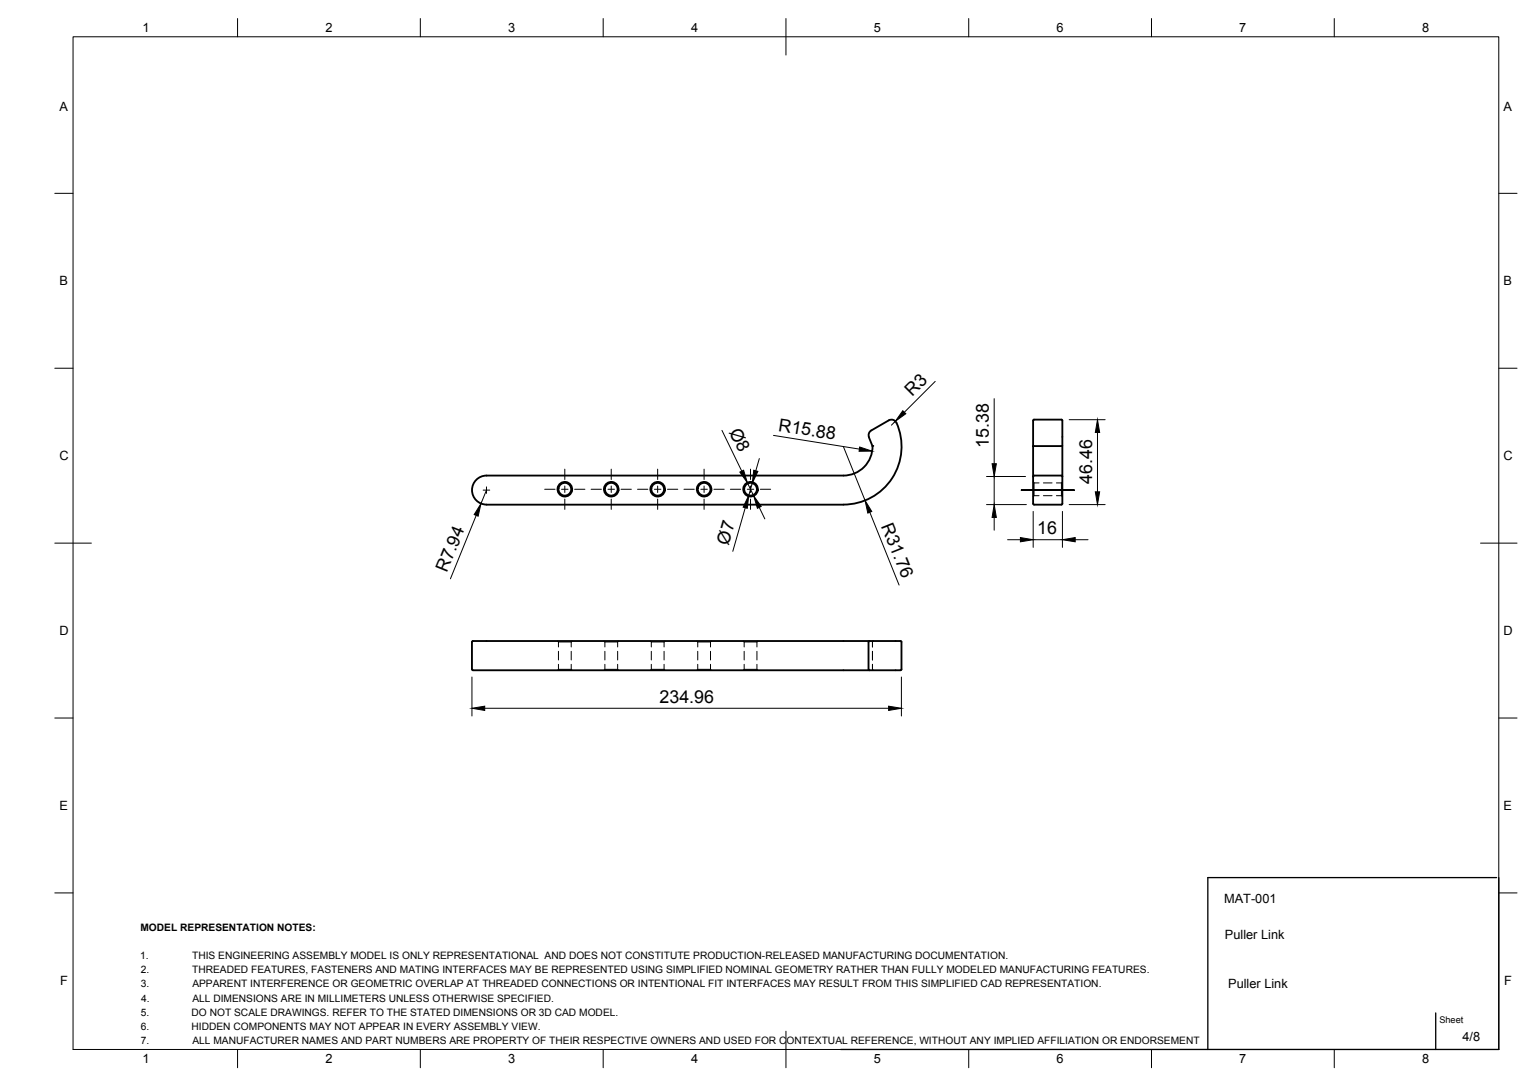
ISO-10303-21;
HEADER;
/* Generated by software containing ST-Developer
 * from STEP Tools, Inc. (www.steptools.com) 
 */

FILE_DESCRIPTION(
/* description */ ('STEP AP214'),
/* implementation_level */ '2;1');

FILE_NAME(
/* name */ 'Puller Link.step',
/* time_stamp */ '2026-11-14T04:30:00-08:00',
/* author */ (''),
/* organization */ (''),
/* preprocessor_version */ 'ST-DEVELOPER v20.2',
/* originating_system */ 'Autodesk Translation Framework v15.17.0.0',
/* authorisation */ '');

FILE_SCHEMA (('AUTOMOTIVE_DESIGN { 1 0 10303 214 3 1 1 }'));
ENDSEC;

DATA;
#10=MECHANICAL_DESIGN_GEOMETRIC_PRESENTATION_REPRESENTATION('',(#130),#40809);
#114=SHAPE_REPRESENTATION_RELATIONSHIP('SRR','None',#40864,#122);
#122=ADVANCED_BREP_SHAPE_REPRESENTATION('',(#138),#40808);
#130=STYLED_ITEM('',(#40906),#138);
#138=MANIFOLD_SOLID_BREP('Body1',#6305);
#329=PLANE('',#7120);
#330=PLANE('',#7124);
#331=PLANE('',#7128);
#332=PLANE('',#7133);
#333=PLANE('',#7134);
#334=PLANE('',#7136);
#359=FACE_BOUND('',#1268,.T.);
#360=FACE_BOUND('',#1269,.T.);
#361=FACE_BOUND('',#1270,.T.);
#362=FACE_BOUND('',#1271,.T.);
#363=FACE_BOUND('',#1272,.T.);
#364=FACE_BOUND('',#1274,.T.);
#365=FACE_BOUND('',#1275,.T.);
#366=FACE_BOUND('',#1276,.T.);
#367=FACE_BOUND('',#1277,.T.);
#368=FACE_BOUND('',#1278,.T.);
#444=CONICAL_SURFACE('',#7074,3.5,0.785398163397436);
#445=CONICAL_SURFACE('',#7078,3.99999999999998,0.785398163397405);
#446=CONICAL_SURFACE('',#7081,3.5,0.785398163397436);
#447=CONICAL_SURFACE('',#7085,4.,0.785398163397429);
#448=CONICAL_SURFACE('',#7088,3.5,0.785398163397436);
#449=CONICAL_SURFACE('',#7092,4.,0.785398163397436);
#450=CONICAL_SURFACE('',#7095,3.49999999999999,0.785398163397435);
#451=CONICAL_SURFACE('',#7099,4.,0.785398163397435);
#452=CONICAL_SURFACE('',#7102,3.49999999999999,0.785398163397435);
#453=CONICAL_SURFACE('',#7106,3.99999999999998,0.785398163397463);
#490=TOROIDAL_SURFACE('',#7056,16.38,0.5);
#491=TOROIDAL_SURFACE('',#7060,31.26,0.5);
#492=TOROIDAL_SURFACE('',#7065,16.38,0.5);
#493=TOROIDAL_SURFACE('',#7069,31.26,0.5);
#494=TOROIDAL_SURFACE('',#7137,2.5,0.5);
#495=TOROIDAL_SURFACE('',#7143,2.5,0.5);
#496=TOROIDAL_SURFACE('',#7145,7.44,0.5);
#497=TOROIDAL_SURFACE('',#7149,2.5,0.5);
#498=TOROIDAL_SURFACE('',#7155,2.5,0.5);
#499=TOROIDAL_SURFACE('',#7157,7.44,0.5);
#839=FACE_OUTER_BOUND('',#1246,.T.);
#840=FACE_OUTER_BOUND('',#1247,.T.);
#841=FACE_OUTER_BOUND('',#1248,.T.);
#842=FACE_OUTER_BOUND('',#1249,.T.);
#843=FACE_OUTER_BOUND('',#1250,.T.);
#844=FACE_OUTER_BOUND('',#1251,.T.);
#845=FACE_OUTER_BOUND('',#1252,.T.);
#846=FACE_OUTER_BOUND('',#1253,.T.);
#847=FACE_OUTER_BOUND('',#1254,.T.);
#848=FACE_OUTER_BOUND('',#1255,.T.);
#849=FACE_OUTER_BOUND('',#1256,.T.);
#850=FACE_OUTER_BOUND('',#1257,.T.);
#851=FACE_OUTER_BOUND('',#1258,.T.);
#852=FACE_OUTER_BOUND('',#1259,.T.);
#853=FACE_OUTER_BOUND('',#1260,.T.);
#854=FACE_OUTER_BOUND('',#1261,.T.);
#855=FACE_OUTER_BOUND('',#1262,.T.);
#856=FACE_OUTER_BOUND('',#1263,.T.);
#857=FACE_OUTER_BOUND('',#1264,.T.);
#858=FACE_OUTER_BOUND('',#1265,.T.);
#859=FACE_OUTER_BOUND('',#1266,.T.);
#860=FACE_OUTER_BOUND('',#1267,.T.);
#861=FACE_OUTER_BOUND('',#1273,.T.);
#862=FACE_OUTER_BOUND('',#1279,.T.);
#863=FACE_OUTER_BOUND('',#1280,.T.);
#864=FACE_OUTER_BOUND('',#1281,.T.);
#865=FACE_OUTER_BOUND('',#1282,.T.);
#866=FACE_OUTER_BOUND('',#1283,.T.);
#867=FACE_OUTER_BOUND('',#1284,.T.);
#868=FACE_OUTER_BOUND('',#1285,.T.);
#869=FACE_OUTER_BOUND('',#1286,.T.);
#870=FACE_OUTER_BOUND('',#1287,.T.);
#871=FACE_OUTER_BOUND('',#1288,.T.);
#872=FACE_OUTER_BOUND('',#1289,.T.);
#873=FACE_OUTER_BOUND('',#1290,.T.);
#874=FACE_OUTER_BOUND('',#1291,.T.);
#875=FACE_OUTER_BOUND('',#1292,.T.);
#876=FACE_OUTER_BOUND('',#1293,.T.);
#877=FACE_OUTER_BOUND('',#1294,.T.);
#878=FACE_OUTER_BOUND('',#1295,.T.);
#879=FACE_OUTER_BOUND('',#1296,.T.);
#880=FACE_OUTER_BOUND('',#1297,.T.);
#881=FACE_OUTER_BOUND('',#1298,.T.);
#882=FACE_OUTER_BOUND('',#1299,.T.);
#1246=EDGE_LOOP('',(#5578,#5579,#5580,#5581));
#1247=EDGE_LOOP('',(#5582,#5583,#5584,#5585));
#1248=EDGE_LOOP('',(#5586,#5587,#5588,#5589));
#1249=EDGE_LOOP('',(#5590,#5591,#5592,#5593));
#1250=EDGE_LOOP('',(#5594,#5595,#5596,#5597,#5598));
#1251=EDGE_LOOP('',(#5599,#5600,#5601,#5602));
#1252=EDGE_LOOP('',(#5603,#5604,#5605,#5606,#5607));
#1253=EDGE_LOOP('',(#5608,#5609,#5610,#5611));
#1254=EDGE_LOOP('',(#5612,#5613,#5614,#5615,#5616));
#1255=EDGE_LOOP('',(#5617,#5618,#5619,#5620));
#1256=EDGE_LOOP('',(#5621,#5622,#5623,#5624,#5625));
#1257=EDGE_LOOP('',(#5626,#5627,#5628,#5629));
#1258=EDGE_LOOP('',(#5630,#5631,#5632,#5633,#5634));
#1259=EDGE_LOOP('',(#5635,#5636,#5637,#5638));
#1260=EDGE_LOOP('',(#5639,#5640,#5641,#5642,#5643));
#1261=EDGE_LOOP('',(#5644,#5645,#5646,#5647,#5648));
#1262=EDGE_LOOP('',(#5649,#5650,#5651,#5652,#5653));
#1263=EDGE_LOOP('',(#5654,#5655,#5656,#5657,#5658));
#1264=EDGE_LOOP('',(#5659,#5660,#5661,#5662,#5663));
#1265=EDGE_LOOP('',(#5664,#5665,#5666,#5667));
#1266=EDGE_LOOP('',(#5668,#5669,#5670,#5671));
#1267=EDGE_LOOP('',(#5672,#5673,#5674,#5675,#5676,#5677,#5678,#5679,#5680));
#1268=EDGE_LOOP('',(#5681));
#1269=EDGE_LOOP('',(#5682));
#1270=EDGE_LOOP('',(#5683));
#1271=EDGE_LOOP('',(#5684));
#1272=EDGE_LOOP('',(#5685));
#1273=EDGE_LOOP('',(#5686,#5687,#5688,#5689,#5690,#5691,#5692,#5693,#5694));
#1274=EDGE_LOOP('',(#5695));
#1275=EDGE_LOOP('',(#5696));
#1276=EDGE_LOOP('',(#5697));
#1277=EDGE_LOOP('',(#5698));
#1278=EDGE_LOOP('',(#5699));
#1279=EDGE_LOOP('',(#5700,#5701,#5702,#5703));
#1280=EDGE_LOOP('',(#5704,#5705,#5706,#5707));
#1281=EDGE_LOOP('',(#5708,#5709,#5710,#5711));
#1282=EDGE_LOOP('',(#5712,#5713,#5714,#5715));
#1283=EDGE_LOOP('',(#5716,#5717,#5718,#5719));
#1284=EDGE_LOOP('',(#5720,#5721,#5722,#5723));
#1285=EDGE_LOOP('',(#5724,#5725,#5726,#5727));
#1286=EDGE_LOOP('',(#5728,#5729,#5730,#5731));
#1287=EDGE_LOOP('',(#5732,#5733,#5734,#5735));
#1288=EDGE_LOOP('',(#5736,#5737,#5738,#5739));
#1289=EDGE_LOOP('',(#5740,#5741,#5742,#5743));
#1290=EDGE_LOOP('',(#5744,#5745,#5746,#5747));
#1291=EDGE_LOOP('',(#5748,#5749,#5750,#5751));
#1292=EDGE_LOOP('',(#5752,#5753,#5754,#5755));
#1293=EDGE_LOOP('',(#5756,#5757,#5758,#5759));
#1294=EDGE_LOOP('',(#5760,#5761,#5762,#5763));
#1295=EDGE_LOOP('',(#5764,#5765,#5766,#5767));
#1296=EDGE_LOOP('',(#5768,#5769,#5770,#5771));
#1297=EDGE_LOOP('',(#5772,#5773,#5774,#5775));
#1298=EDGE_LOOP('',(#5776,#5777,#5778,#5779));
#1299=EDGE_LOOP('',(#5780,#5781,#5782,#5783));
#1639=CIRCLE('',#7057,16.38);
#1640=CIRCLE('',#7058,15.88);
#1641=CIRCLE('',#7059,0.5);
#1642=CIRCLE('',#7061,31.76);
#1643=CIRCLE('',#7062,0.500000000000001);
#1644=CIRCLE('',#7063,31.26);
#1645=CIRCLE('',#7064,0.5);
#1646=CIRCLE('',#7066,15.88);
#1647=CIRCLE('',#7067,16.38);
#1648=CIRCLE('',#7068,0.5);
#1649=CIRCLE('',#7070,31.26);
#1650=CIRCLE('',#7071,0.500000000000001);
#1651=CIRCLE('',#7072,31.76);
#1652=CIRCLE('',#7073,0.5);
#1653=CIRCLE('',#7075,3.5);
#1654=CIRCLE('',#7076,3.5);
#1655=CIRCLE('',#7077,4.00000000000003);
#1656=CIRCLE('',#7079,3.5);
#1657=CIRCLE('',#7080,3.99999999999998);
#1658=CIRCLE('',#7082,3.5);
#1659=CIRCLE('',#7083,3.5);
#1660=CIRCLE('',#7084,4.00000000000003);
#1661=CIRCLE('',#7086,3.5);
#1662=CIRCLE('',#7087,4.);
#1663=CIRCLE('',#7089,3.5);
#1664=CIRCLE('',#7090,3.5);
#1665=CIRCLE('',#7091,4.00000000000003);
#1666=CIRCLE('',#7093,3.5);
#1667=CIRCLE('',#7094,4.);
#1668=CIRCLE('',#7096,3.49999999999999);
#1669=CIRCLE('',#7097,3.49999999999999);
#1670=CIRCLE('',#7098,4.00000000000003);
#1671=CIRCLE('',#7100,3.49999999999999);
#1672=CIRCLE('',#7101,4.);
#1673=CIRCLE('',#7103,3.49999999999999);
#1674=CIRCLE('',#7104,3.49999999999999);
#1675=CIRCLE('',#7105,4.00000000000003);
#1676=CIRCLE('',#7107,3.49999999999999);
#1677=CIRCLE('',#7108,3.99999999999998);
#1678=CIRCLE('',#7115,3.);
#1679=CIRCLE('',#7116,3.);
#1680=CIRCLE('',#7118,7.94);
#1681=CIRCLE('',#7119,7.94);
#1682=CIRCLE('',#7121,7.44);
#1683=CIRCLE('',#7122,2.5);
#1684=CIRCLE('',#7123,2.5);
#1685=CIRCLE('',#7125,2.5);
#1686=CIRCLE('',#7126,2.5);
#1687=CIRCLE('',#7127,7.44);
#1688=CIRCLE('',#7131,3.);
#1689=CIRCLE('',#7132,3.);
#1690=CIRCLE('',#7138,0.500000000000002);
#1691=CIRCLE('',#7140,0.500000000000002);
#1692=CIRCLE('',#7142,0.5);
#1693=CIRCLE('',#7144,0.499999999999993);
#1694=CIRCLE('',#7146,0.5);
#1695=CIRCLE('',#7150,0.500000000000002);
#1696=CIRCLE('',#7152,0.500000000000002);
#1697=CIRCLE('',#7154,0.5);
#1698=CIRCLE('',#7156,0.499999999999992);
#1699=CIRCLE('',#7158,0.5);
#1825=B_SPLINE_CURVE_WITH_KNOTS('',3,(#40537,#40538,#40539,#40540,#40541,
#40542,#40543,#40544,#40545,#40546,#40547,#40548,#40549,#40550),
 .UNSPECIFIED.,.F.,.F.,(4,2,2,2,2,2,4),(-0.158545503402535,-0.158223124815241,
-0.138074238874086,-0.118093212716543,-0.0984509148305753,-0.0791141254766957,
-0.0790886006090571),.UNSPECIFIED.);
#1826=B_SPLINE_CURVE_WITH_KNOTS('',3,(#40568,#40569,#40570,#40571,#40572,
#40573,#40574,#40575,#40576,#40577,#40578,#40579,#40580,#40581),
 .UNSPECIFIED.,.F.,.F.,(4,2,2,2,2,2,4),(-0.0791417248593108,-0.0791161976751982,
-0.059777648817268,-0.0401335636282681,-0.0201507193459134,-2.01783034725622E-14,
0.000322407921445618),.UNSPECIFIED.);
#2105=LINE('',#40600,#2423);
#2106=LINE('',#40606,#2424);
#2107=LINE('',#40614,#2425);
#2108=LINE('',#40620,#2426);
#2109=LINE('',#40628,#2427);
#2110=LINE('',#40634,#2428);
#2111=LINE('',#40642,#2429);
#2112=LINE('',#40648,#2430);
#2113=LINE('',#40656,#2431);
#2114=LINE('',#40662,#2432);
#2115=LINE('',#40665,#2433);
#2116=LINE('',#40667,#2434);
#2117=LINE('',#40669,#2435);
#2118=LINE('',#40671,#2436);
#2119=LINE('',#40673,#2437);
#2120=LINE('',#40679,#2438);
#2121=LINE('',#40682,#2439);
#2122=LINE('',#40688,#2440);
#2123=LINE('',#40691,#2441);
#2124=LINE('',#40694,#2442);
#2125=LINE('',#40696,#2443);
#2126=LINE('',#40699,#2444);
#2127=LINE('',#40703,#2445);
#2128=LINE('',#40707,#2446);
#2129=LINE('',#40709,#2447);
#2130=LINE('',#40713,#2448);
#2131=LINE('',#40716,#2449);
#2132=LINE('',#40719,#2450);
#2133=LINE('',#40720,#2451);
#2134=LINE('',#40721,#2452);
#2135=LINE('',#40723,#2453);
#2136=LINE('',#40728,#2454);
#2137=LINE('',#40731,#2455);
#2138=LINE('',#40732,#2456);
#2139=LINE('',#40734,#2457);
#2140=LINE('',#40735,#2458);
#2141=LINE('',#40736,#2459);
#2142=LINE('',#40738,#2460);
#2143=LINE('',#40740,#2461);
#2144=LINE('',#40741,#2462);
#2423=VECTOR('',#8827,3.5);
#2424=VECTOR('',#8834,3.99999999999998);
#2425=VECTOR('',#8843,3.5);
#2426=VECTOR('',#8850,4.);
#2427=VECTOR('',#8859,3.5);
#2428=VECTOR('',#8866,4.);
#2429=VECTOR('',#8875,3.49999999999999);
#2430=VECTOR('',#8882,4.);
#2431=VECTOR('',#8891,3.49999999999999);
#2432=VECTOR('',#8898,3.99999999999998);
#2433=VECTOR('',#8903,3.49999999999999);
#2434=VECTOR('',#8906,3.49999999999999);
#2435=VECTOR('',#8909,3.5);
#2436=VECTOR('',#8912,3.5);
#2437=VECTOR('',#8915,3.5);
#2438=VECTOR('',#8920,1000.);
#2439=VECTOR('',#8923,1000.);
#2440=VECTOR('',#8928,1000.);
#2441=VECTOR('',#8931,1000.);
#2442=VECTOR('',#8934,1000.);
#2443=VECTOR('',#8935,1000.);
#2444=VECTOR('',#8938,1000.);
#2445=VECTOR('',#8941,1000.);
#2446=VECTOR('',#8946,1000.);
#2447=VECTOR('',#8947,1000.);
#2448=VECTOR('',#8950,1000.);
#2449=VECTOR('',#8953,1000.);
#2450=VECTOR('',#8958,1000.);
#2451=VECTOR('',#8959,1000.);
#2452=VECTOR('',#8960,1000.);
#2453=VECTOR('',#8963,1000.);
#2454=VECTOR('',#8968,1000.);
#2455=VECTOR('',#8973,1000.);
#2456=VECTOR('',#8974,1000.);
#2457=VECTOR('',#8977,1000.);
#2458=VECTOR('',#8978,1000.);
#2459=VECTOR('',#8979,1000.);
#2460=VECTOR('',#8982,1000.);
#2461=VECTOR('',#8985,1000.);
#2462=VECTOR('',#8986,1000.);
#2963=VERTEX_POINT('',#40533);
#2964=VERTEX_POINT('',#40534);
#2965=VERTEX_POINT('',#40536);
#2966=VERTEX_POINT('',#40551);
#2967=VERTEX_POINT('',#40555);
#2968=VERTEX_POINT('',#40556);
#2969=VERTEX_POINT('',#40558);
#2970=VERTEX_POINT('',#40560);
#2971=VERTEX_POINT('',#40564);
#2972=VERTEX_POINT('',#40565);
#2973=VERTEX_POINT('',#40567);
#2974=VERTEX_POINT('',#40582);
#2975=VERTEX_POINT('',#40586);
#2976=VERTEX_POINT('',#40587);
#2977=VERTEX_POINT('',#40589);
#2978=VERTEX_POINT('',#40591);
#2979=VERTEX_POINT('',#40595);
#2980=VERTEX_POINT('',#40596);
#2981=VERTEX_POINT('',#40599);
#2982=VERTEX_POINT('',#40603);
#2983=VERTEX_POINT('',#40605);
#2984=VERTEX_POINT('',#40609);
#2985=VERTEX_POINT('',#40610);
#2986=VERTEX_POINT('',#40613);
#2987=VERTEX_POINT('',#40617);
#2988=VERTEX_POINT('',#40619);
#2989=VERTEX_POINT('',#40623);
#2990=VERTEX_POINT('',#40624);
#2991=VERTEX_POINT('',#40627);
#2992=VERTEX_POINT('',#40631);
#2993=VERTEX_POINT('',#40633);
#2994=VERTEX_POINT('',#40637);
#2995=VERTEX_POINT('',#40638);
#2996=VERTEX_POINT('',#40641);
#2997=VERTEX_POINT('',#40645);
#2998=VERTEX_POINT('',#40647);
#2999=VERTEX_POINT('',#40651);
#3000=VERTEX_POINT('',#40652);
#3001=VERTEX_POINT('',#40655);
#3002=VERTEX_POINT('',#40659);
#3003=VERTEX_POINT('',#40661);
#3004=VERTEX_POINT('',#40675);
#3005=VERTEX_POINT('',#40676);
#3006=VERTEX_POINT('',#40678);
#3007=VERTEX_POINT('',#40680);
#3008=VERTEX_POINT('',#40684);
#3009=VERTEX_POINT('',#40685);
#3010=VERTEX_POINT('',#40687);
#3011=VERTEX_POINT('',#40689);
#3012=VERTEX_POINT('',#40693);
#3013=VERTEX_POINT('',#40695);
#3014=VERTEX_POINT('',#40697);
#3015=VERTEX_POINT('',#40700);
#3016=VERTEX_POINT('',#40702);
#3017=VERTEX_POINT('',#40706);
#3018=VERTEX_POINT('',#40708);
#3019=VERTEX_POINT('',#40710);
#3020=VERTEX_POINT('',#40712);
#3021=VERTEX_POINT('',#40715);
#3022=VERTEX_POINT('',#40725);
#3023=VERTEX_POINT('',#40727);
#3841=EDGE_CURVE('',#2963,#2964,#1639,.T.);
#3842=EDGE_CURVE('',#2963,#2965,#1825,.T.);
#3843=EDGE_CURVE('',#2966,#2965,#1640,.T.);
#3844=EDGE_CURVE('',#2966,#2964,#1641,.T.);
#3845=EDGE_CURVE('',#2967,#2968,#1642,.T.);
#3846=EDGE_CURVE('',#2967,#2969,#1643,.T.);
#3847=EDGE_CURVE('',#2970,#2969,#1644,.T.);
#3848=EDGE_CURVE('',#2968,#2970,#1645,.T.);
#3849=EDGE_CURVE('',#2971,#2972,#1646,.T.);
#3850=EDGE_CURVE('',#2971,#2973,#1826,.T.);
#3851=EDGE_CURVE('',#2974,#2973,#1647,.T.);
#3852=EDGE_CURVE('',#2974,#2972,#1648,.T.);
#3853=EDGE_CURVE('',#2975,#2976,#1649,.T.);
#3854=EDGE_CURVE('',#2975,#2977,#1650,.T.);
#3855=EDGE_CURVE('',#2978,#2977,#1651,.T.);
#3856=EDGE_CURVE('',#2976,#2978,#1652,.T.);
#3857=EDGE_CURVE('',#2979,#2980,#1653,.T.);
#3858=EDGE_CURVE('',#2980,#2979,#1654,.T.);
#3859=EDGE_CURVE('',#2980,#2981,#2105,.T.);
#3860=EDGE_CURVE('',#2981,#2981,#1655,.T.);
#3861=EDGE_CURVE('',#2982,#2982,#1656,.T.);
#3862=EDGE_CURVE('',#2982,#2983,#2106,.T.);
#3863=EDGE_CURVE('',#2983,#2983,#1657,.T.);
#3864=EDGE_CURVE('',#2984,#2985,#1658,.T.);
#3865=EDGE_CURVE('',#2985,#2984,#1659,.T.);
#3866=EDGE_CURVE('',#2985,#2986,#2107,.T.);
#3867=EDGE_CURVE('',#2986,#2986,#1660,.T.);
#3868=EDGE_CURVE('',#2987,#2987,#1661,.T.);
#3869=EDGE_CURVE('',#2987,#2988,#2108,.T.);
#3870=EDGE_CURVE('',#2988,#2988,#1662,.T.);
#3871=EDGE_CURVE('',#2989,#2990,#1663,.T.);
#3872=EDGE_CURVE('',#2990,#2989,#1664,.T.);
#3873=EDGE_CURVE('',#2990,#2991,#2109,.T.);
#3874=EDGE_CURVE('',#2991,#2991,#1665,.T.);
#3875=EDGE_CURVE('',#2992,#2992,#1666,.T.);
#3876=EDGE_CURVE('',#2992,#2993,#2110,.T.);
#3877=EDGE_CURVE('',#2993,#2993,#1667,.T.);
#3878=EDGE_CURVE('',#2994,#2995,#1668,.T.);
#3879=EDGE_CURVE('',#2995,#2994,#1669,.T.);
#3880=EDGE_CURVE('',#2995,#2996,#2111,.T.);
#3881=EDGE_CURVE('',#2996,#2996,#1670,.T.);
#3882=EDGE_CURVE('',#2997,#2997,#1671,.T.);
#3883=EDGE_CURVE('',#2997,#2998,#2112,.T.);
#3884=EDGE_CURVE('',#2998,#2998,#1672,.T.);
#3885=EDGE_CURVE('',#2999,#3000,#1673,.T.);
#3886=EDGE_CURVE('',#3000,#2999,#1674,.T.);
#3887=EDGE_CURVE('',#3000,#3001,#2113,.T.);
#3888=EDGE_CURVE('',#3001,#3001,#1675,.T.);
#3889=EDGE_CURVE('',#3002,#3002,#1676,.T.);
#3890=EDGE_CURVE('',#3002,#3003,#2114,.T.);
#3891=EDGE_CURVE('',#3003,#3003,#1677,.T.);
#3892=EDGE_CURVE('',#2999,#3002,#2115,.T.);
#3893=EDGE_CURVE('',#2994,#2997,#2116,.T.);
#3894=EDGE_CURVE('',#2989,#2992,#2117,.T.);
#3895=EDGE_CURVE('',#2984,#2987,#2118,.T.);
#3896=EDGE_CURVE('',#2979,#2982,#2119,.T.);
#3897=EDGE_CURVE('',#3004,#3005,#1678,.T.);
#3898=EDGE_CURVE('',#3005,#3006,#2120,.T.);
#3899=EDGE_CURVE('',#3006,#3007,#1679,.T.);
#3900=EDGE_CURVE('',#3004,#3007,#2121,.T.);
#3901=EDGE_CURVE('',#3008,#3009,#1680,.T.);
#3902=EDGE_CURVE('',#3009,#3010,#2122,.T.);
#3903=EDGE_CURVE('',#3010,#3011,#1681,.T.);
#3904=EDGE_CURVE('',#3008,#3011,#2123,.T.);
#3905=EDGE_CURVE('',#3012,#2963,#2124,.T.);
#3906=EDGE_CURVE('',#2964,#3013,#2125,.T.);
#3907=EDGE_CURVE('',#3013,#3014,#1682,.T.);
#3908=EDGE_CURVE('',#3014,#2970,#2126,.T.);
#3909=EDGE_CURVE('',#2969,#3015,#1683,.T.);
#3910=EDGE_CURVE('',#3015,#3016,#2127,.T.);
#3911=EDGE_CURVE('',#3016,#3012,#1684,.T.);
#3912=EDGE_CURVE('',#3017,#2974,#2128,.T.);
#3913=EDGE_CURVE('',#2973,#3018,#2129,.T.);
#3914=EDGE_CURVE('',#3018,#3019,#1685,.T.);
#3915=EDGE_CURVE('',#3019,#3020,#2130,.T.);
#3916=EDGE_CURVE('',#3020,#2975,#1686,.T.);
#3917=EDGE_CURVE('',#2976,#3021,#2131,.T.);
#3918=EDGE_CURVE('',#3021,#3017,#1687,.T.);
#3919=EDGE_CURVE('',#2968,#2978,#2132,.T.);
#3920=EDGE_CURVE('',#2968,#3008,#2133,.T.);
#3921=EDGE_CURVE('',#3011,#2978,#2134,.T.);
#3922=EDGE_CURVE('',#2967,#2977,#2135,.T.);
#3923=EDGE_CURVE('',#2977,#3022,#1688,.T.);
#3924=EDGE_CURVE('',#3023,#3022,#2136,.T.);
#3925=EDGE_CURVE('',#3023,#2967,#1689,.T.);
#3926=EDGE_CURVE('',#3022,#3006,#2137,.T.);
#3927=EDGE_CURVE('',#3005,#3023,#2138,.T.);
#3928=EDGE_CURVE('',#3007,#2971,#2139,.T.);
#3929=EDGE_CURVE('',#2965,#2971,#2140,.T.);
#3930=EDGE_CURVE('',#2965,#3004,#2141,.T.);
#3931=EDGE_CURVE('',#2966,#2972,#2142,.T.);
#3932=EDGE_CURVE('',#2972,#3010,#2143,.T.);
#3933=EDGE_CURVE('',#3009,#2966,#2144,.T.);
#3934=EDGE_CURVE('',#3022,#3020,#1690,.T.);
#3935=EDGE_CURVE('',#3006,#3019,#1691,.T.);
#3936=EDGE_CURVE('',#3021,#3011,#1692,.T.);
#3937=EDGE_CURVE('',#3007,#3018,#1693,.T.);
#3938=EDGE_CURVE('',#3017,#3010,#1694,.T.);
#3939=EDGE_CURVE('',#3015,#3023,#1695,.T.);
#3940=EDGE_CURVE('',#3016,#3005,#1696,.T.);
#3941=EDGE_CURVE('',#3008,#3014,#1697,.T.);
#3942=EDGE_CURVE('',#3012,#3004,#1698,.T.);
#3943=EDGE_CURVE('',#3009,#3013,#1699,.T.);
#5578=ORIENTED_EDGE('',*,*,#3841,.F.);
#5579=ORIENTED_EDGE('',*,*,#3842,.T.);
#5580=ORIENTED_EDGE('',*,*,#3843,.F.);
#5581=ORIENTED_EDGE('',*,*,#3844,.T.);
#5582=ORIENTED_EDGE('',*,*,#3845,.F.);
#5583=ORIENTED_EDGE('',*,*,#3846,.T.);
#5584=ORIENTED_EDGE('',*,*,#3847,.F.);
#5585=ORIENTED_EDGE('',*,*,#3848,.F.);
#5586=ORIENTED_EDGE('',*,*,#3849,.F.);
#5587=ORIENTED_EDGE('',*,*,#3850,.T.);
#5588=ORIENTED_EDGE('',*,*,#3851,.F.);
#5589=ORIENTED_EDGE('',*,*,#3852,.T.);
#5590=ORIENTED_EDGE('',*,*,#3853,.F.);
#5591=ORIENTED_EDGE('',*,*,#3854,.T.);
#5592=ORIENTED_EDGE('',*,*,#3855,.F.);
#5593=ORIENTED_EDGE('',*,*,#3856,.F.);
#5594=ORIENTED_EDGE('',*,*,#3857,.F.);
#5595=ORIENTED_EDGE('',*,*,#3858,.F.);
#5596=ORIENTED_EDGE('',*,*,#3859,.T.);
#5597=ORIENTED_EDGE('',*,*,#3860,.F.);
#5598=ORIENTED_EDGE('',*,*,#3859,.F.);
#5599=ORIENTED_EDGE('',*,*,#3861,.F.);
#5600=ORIENTED_EDGE('',*,*,#3862,.T.);
#5601=ORIENTED_EDGE('',*,*,#3863,.F.);
#5602=ORIENTED_EDGE('',*,*,#3862,.F.);
#5603=ORIENTED_EDGE('',*,*,#3864,.F.);
#5604=ORIENTED_EDGE('',*,*,#3865,.F.);
#5605=ORIENTED_EDGE('',*,*,#3866,.T.);
#5606=ORIENTED_EDGE('',*,*,#3867,.F.);
#5607=ORIENTED_EDGE('',*,*,#3866,.F.);
#5608=ORIENTED_EDGE('',*,*,#3868,.F.);
#5609=ORIENTED_EDGE('',*,*,#3869,.T.);
#5610=ORIENTED_EDGE('',*,*,#3870,.F.);
#5611=ORIENTED_EDGE('',*,*,#3869,.F.);
#5612=ORIENTED_EDGE('',*,*,#3871,.F.);
#5613=ORIENTED_EDGE('',*,*,#3872,.F.);
#5614=ORIENTED_EDGE('',*,*,#3873,.T.);
#5615=ORIENTED_EDGE('',*,*,#3874,.F.);
#5616=ORIENTED_EDGE('',*,*,#3873,.F.);
#5617=ORIENTED_EDGE('',*,*,#3875,.F.);
#5618=ORIENTED_EDGE('',*,*,#3876,.T.);
#5619=ORIENTED_EDGE('',*,*,#3877,.F.);
#5620=ORIENTED_EDGE('',*,*,#3876,.F.);
#5621=ORIENTED_EDGE('',*,*,#3878,.F.);
#5622=ORIENTED_EDGE('',*,*,#3879,.F.);
#5623=ORIENTED_EDGE('',*,*,#3880,.T.);
#5624=ORIENTED_EDGE('',*,*,#3881,.F.);
#5625=ORIENTED_EDGE('',*,*,#3880,.F.);
#5626=ORIENTED_EDGE('',*,*,#3882,.F.);
#5627=ORIENTED_EDGE('',*,*,#3883,.T.);
#5628=ORIENTED_EDGE('',*,*,#3884,.F.);
#5629=ORIENTED_EDGE('',*,*,#3883,.F.);
#5630=ORIENTED_EDGE('',*,*,#3885,.F.);
#5631=ORIENTED_EDGE('',*,*,#3886,.F.);
#5632=ORIENTED_EDGE('',*,*,#3887,.T.);
#5633=ORIENTED_EDGE('',*,*,#3888,.F.);
#5634=ORIENTED_EDGE('',*,*,#3887,.F.);
#5635=ORIENTED_EDGE('',*,*,#3889,.F.);
#5636=ORIENTED_EDGE('',*,*,#3890,.T.);
#5637=ORIENTED_EDGE('',*,*,#3891,.F.);
#5638=ORIENTED_EDGE('',*,*,#3890,.F.);
#5639=ORIENTED_EDGE('',*,*,#3885,.T.);
#5640=ORIENTED_EDGE('',*,*,#3886,.T.);
#5641=ORIENTED_EDGE('',*,*,#3892,.T.);
#5642=ORIENTED_EDGE('',*,*,#3889,.T.);
#5643=ORIENTED_EDGE('',*,*,#3892,.F.);
#5644=ORIENTED_EDGE('',*,*,#3878,.T.);
#5645=ORIENTED_EDGE('',*,*,#3879,.T.);
#5646=ORIENTED_EDGE('',*,*,#3893,.T.);
#5647=ORIENTED_EDGE('',*,*,#3882,.T.);
#5648=ORIENTED_EDGE('',*,*,#3893,.F.);
#5649=ORIENTED_EDGE('',*,*,#3871,.T.);
#5650=ORIENTED_EDGE('',*,*,#3872,.T.);
#5651=ORIENTED_EDGE('',*,*,#3894,.T.);
#5652=ORIENTED_EDGE('',*,*,#3875,.T.);
#5653=ORIENTED_EDGE('',*,*,#3894,.F.);
#5654=ORIENTED_EDGE('',*,*,#3864,.T.);
#5655=ORIENTED_EDGE('',*,*,#3865,.T.);
#5656=ORIENTED_EDGE('',*,*,#3895,.T.);
#5657=ORIENTED_EDGE('',*,*,#3868,.T.);
#5658=ORIENTED_EDGE('',*,*,#3895,.F.);
#5659=ORIENTED_EDGE('',*,*,#3857,.T.);
#5660=ORIENTED_EDGE('',*,*,#3858,.T.);
#5661=ORIENTED_EDGE('',*,*,#3896,.T.);
#5662=ORIENTED_EDGE('',*,*,#3861,.T.);
#5663=ORIENTED_EDGE('',*,*,#3896,.F.);
#5664=ORIENTED_EDGE('',*,*,#3897,.T.);
#5665=ORIENTED_EDGE('',*,*,#3898,.T.);
#5666=ORIENTED_EDGE('',*,*,#3899,.T.);
#5667=ORIENTED_EDGE('',*,*,#3900,.F.);
#5668=ORIENTED_EDGE('',*,*,#3901,.T.);
#5669=ORIENTED_EDGE('',*,*,#3902,.T.);
#5670=ORIENTED_EDGE('',*,*,#3903,.T.);
#5671=ORIENTED_EDGE('',*,*,#3904,.F.);
#5672=ORIENTED_EDGE('',*,*,#3905,.T.);
#5673=ORIENTED_EDGE('',*,*,#3841,.T.);
#5674=ORIENTED_EDGE('',*,*,#3906,.T.);
#5675=ORIENTED_EDGE('',*,*,#3907,.T.);
#5676=ORIENTED_EDGE('',*,*,#3908,.T.);
#5677=ORIENTED_EDGE('',*,*,#3847,.T.);
#5678=ORIENTED_EDGE('',*,*,#3909,.T.);
#5679=ORIENTED_EDGE('',*,*,#3910,.T.);
#5680=ORIENTED_EDGE('',*,*,#3911,.T.);
#5681=ORIENTED_EDGE('',*,*,#3888,.T.);
#5682=ORIENTED_EDGE('',*,*,#3881,.T.);
#5683=ORIENTED_EDGE('',*,*,#3874,.T.);
#5684=ORIENTED_EDGE('',*,*,#3867,.T.);
#5685=ORIENTED_EDGE('',*,*,#3860,.T.);
#5686=ORIENTED_EDGE('',*,*,#3912,.T.);
#5687=ORIENTED_EDGE('',*,*,#3851,.T.);
#5688=ORIENTED_EDGE('',*,*,#3913,.T.);
#5689=ORIENTED_EDGE('',*,*,#3914,.T.);
#5690=ORIENTED_EDGE('',*,*,#3915,.T.);
#5691=ORIENTED_EDGE('',*,*,#3916,.T.);
#5692=ORIENTED_EDGE('',*,*,#3853,.T.);
#5693=ORIENTED_EDGE('',*,*,#3917,.T.);
#5694=ORIENTED_EDGE('',*,*,#3918,.T.);
#5695=ORIENTED_EDGE('',*,*,#3891,.T.);
#5696=ORIENTED_EDGE('',*,*,#3884,.T.);
#5697=ORIENTED_EDGE('',*,*,#3877,.T.);
#5698=ORIENTED_EDGE('',*,*,#3870,.T.);
#5699=ORIENTED_EDGE('',*,*,#3863,.T.);
#5700=ORIENTED_EDGE('',*,*,#3919,.F.);
#5701=ORIENTED_EDGE('',*,*,#3920,.T.);
#5702=ORIENTED_EDGE('',*,*,#3904,.T.);
#5703=ORIENTED_EDGE('',*,*,#3921,.T.);
#5704=ORIENTED_EDGE('',*,*,#3919,.T.);
#5705=ORIENTED_EDGE('',*,*,#3855,.T.);
#5706=ORIENTED_EDGE('',*,*,#3922,.F.);
#5707=ORIENTED_EDGE('',*,*,#3845,.T.);
#5708=ORIENTED_EDGE('',*,*,#3922,.T.);
#5709=ORIENTED_EDGE('',*,*,#3923,.T.);
#5710=ORIENTED_EDGE('',*,*,#3924,.F.);
#5711=ORIENTED_EDGE('',*,*,#3925,.T.);
#5712=ORIENTED_EDGE('',*,*,#3924,.T.);
#5713=ORIENTED_EDGE('',*,*,#3926,.T.);
#5714=ORIENTED_EDGE('',*,*,#3898,.F.);
#5715=ORIENTED_EDGE('',*,*,#3927,.T.);
#5716=ORIENTED_EDGE('',*,*,#3900,.T.);
#5717=ORIENTED_EDGE('',*,*,#3928,.T.);
#5718=ORIENTED_EDGE('',*,*,#3929,.F.);
#5719=ORIENTED_EDGE('',*,*,#3930,.T.);
#5720=ORIENTED_EDGE('',*,*,#3929,.T.);
#5721=ORIENTED_EDGE('',*,*,#3849,.T.);
#5722=ORIENTED_EDGE('',*,*,#3931,.F.);
#5723=ORIENTED_EDGE('',*,*,#3843,.T.);
#5724=ORIENTED_EDGE('',*,*,#3931,.T.);
#5725=ORIENTED_EDGE('',*,*,#3932,.T.);
#5726=ORIENTED_EDGE('',*,*,#3902,.F.);
#5727=ORIENTED_EDGE('',*,*,#3933,.T.);
#5728=ORIENTED_EDGE('',*,*,#3934,.F.);
#5729=ORIENTED_EDGE('',*,*,#3923,.F.);
#5730=ORIENTED_EDGE('',*,*,#3854,.F.);
#5731=ORIENTED_EDGE('',*,*,#3916,.F.);
#5732=ORIENTED_EDGE('',*,*,#3934,.T.);
#5733=ORIENTED_EDGE('',*,*,#3915,.F.);
#5734=ORIENTED_EDGE('',*,*,#3935,.F.);
#5735=ORIENTED_EDGE('',*,*,#3926,.F.);
#5736=ORIENTED_EDGE('',*,*,#3856,.T.);
#5737=ORIENTED_EDGE('',*,*,#3921,.F.);
#5738=ORIENTED_EDGE('',*,*,#3936,.F.);
#5739=ORIENTED_EDGE('',*,*,#3917,.F.);
#5740=ORIENTED_EDGE('',*,*,#3935,.T.);
#5741=ORIENTED_EDGE('',*,*,#3914,.F.);
#5742=ORIENTED_EDGE('',*,*,#3937,.F.);
#5743=ORIENTED_EDGE('',*,*,#3899,.F.);
#5744=ORIENTED_EDGE('',*,*,#3936,.T.);
#5745=ORIENTED_EDGE('',*,*,#3903,.F.);
#5746=ORIENTED_EDGE('',*,*,#3938,.F.);
#5747=ORIENTED_EDGE('',*,*,#3918,.F.);
#5748=ORIENTED_EDGE('',*,*,#3937,.T.);
#5749=ORIENTED_EDGE('',*,*,#3913,.F.);
#5750=ORIENTED_EDGE('',*,*,#3850,.F.);
#5751=ORIENTED_EDGE('',*,*,#3928,.F.);
#5752=ORIENTED_EDGE('',*,*,#3938,.T.);
#5753=ORIENTED_EDGE('',*,*,#3932,.F.);
#5754=ORIENTED_EDGE('',*,*,#3852,.F.);
#5755=ORIENTED_EDGE('',*,*,#3912,.F.);
#5756=ORIENTED_EDGE('',*,*,#3939,.F.);
#5757=ORIENTED_EDGE('',*,*,#3909,.F.);
#5758=ORIENTED_EDGE('',*,*,#3846,.F.);
#5759=ORIENTED_EDGE('',*,*,#3925,.F.);
#5760=ORIENTED_EDGE('',*,*,#3939,.T.);
#5761=ORIENTED_EDGE('',*,*,#3927,.F.);
#5762=ORIENTED_EDGE('',*,*,#3940,.F.);
#5763=ORIENTED_EDGE('',*,*,#3910,.F.);
#5764=ORIENTED_EDGE('',*,*,#3848,.T.);
#5765=ORIENTED_EDGE('',*,*,#3908,.F.);
#5766=ORIENTED_EDGE('',*,*,#3941,.F.);
#5767=ORIENTED_EDGE('',*,*,#3920,.F.);
#5768=ORIENTED_EDGE('',*,*,#3940,.T.);
#5769=ORIENTED_EDGE('',*,*,#3897,.F.);
#5770=ORIENTED_EDGE('',*,*,#3942,.F.);
#5771=ORIENTED_EDGE('',*,*,#3911,.F.);
#5772=ORIENTED_EDGE('',*,*,#3941,.T.);
#5773=ORIENTED_EDGE('',*,*,#3907,.F.);
#5774=ORIENTED_EDGE('',*,*,#3943,.F.);
#5775=ORIENTED_EDGE('',*,*,#3901,.F.);
#5776=ORIENTED_EDGE('',*,*,#3942,.T.);
#5777=ORIENTED_EDGE('',*,*,#3930,.F.);
#5778=ORIENTED_EDGE('',*,*,#3842,.F.);
#5779=ORIENTED_EDGE('',*,*,#3905,.F.);
#5780=ORIENTED_EDGE('',*,*,#3943,.T.);
#5781=ORIENTED_EDGE('',*,*,#3906,.F.);
#5782=ORIENTED_EDGE('',*,*,#3844,.F.);
#5783=ORIENTED_EDGE('',*,*,#3933,.F.);
#5897=CYLINDRICAL_SURFACE('',#7109,3.49999999999999);
#5898=CYLINDRICAL_SURFACE('',#7110,3.49999999999999);
#5899=CYLINDRICAL_SURFACE('',#7111,3.5);
#5900=CYLINDRICAL_SURFACE('',#7112,3.5);
#5901=CYLINDRICAL_SURFACE('',#7113,3.5);
#5902=CYLINDRICAL_SURFACE('',#7114,3.);
#5903=CYLINDRICAL_SURFACE('',#7117,7.94);
#5904=CYLINDRICAL_SURFACE('',#7129,31.76);
#5905=CYLINDRICAL_SURFACE('',#7130,3.);
#5906=CYLINDRICAL_SURFACE('',#7135,15.88);
#5907=CYLINDRICAL_SURFACE('',#7139,0.500000000000002);
#5908=CYLINDRICAL_SURFACE('',#7141,0.5);
#5909=CYLINDRICAL_SURFACE('',#7147,0.499999999999991);
#5910=CYLINDRICAL_SURFACE('',#7148,0.5);
#5911=CYLINDRICAL_SURFACE('',#7151,0.500000000000002);
#5912=CYLINDRICAL_SURFACE('',#7153,0.5);
#5913=CYLINDRICAL_SURFACE('',#7159,0.499999999999989);
#5914=CYLINDRICAL_SURFACE('',#7160,0.5);
#6254=ADVANCED_FACE('',(#839),#490,.T.);
#6255=ADVANCED_FACE('',(#840),#491,.T.);
#6256=ADVANCED_FACE('',(#841),#492,.T.);
#6257=ADVANCED_FACE('',(#842),#493,.T.);
#6258=ADVANCED_FACE('',(#843),#444,.F.);
#6259=ADVANCED_FACE('',(#844),#445,.F.);
#6260=ADVANCED_FACE('',(#845),#446,.F.);
#6261=ADVANCED_FACE('',(#846),#447,.F.);
#6262=ADVANCED_FACE('',(#847),#448,.F.);
#6263=ADVANCED_FACE('',(#848),#449,.F.);
#6264=ADVANCED_FACE('',(#849),#450,.F.);
#6265=ADVANCED_FACE('',(#850),#451,.F.);
#6266=ADVANCED_FACE('',(#851),#452,.F.);
#6267=ADVANCED_FACE('',(#852),#453,.F.);
#6268=ADVANCED_FACE('',(#853),#5897,.F.);
#6269=ADVANCED_FACE('',(#854),#5898,.F.);
#6270=ADVANCED_FACE('',(#855),#5899,.F.);
#6271=ADVANCED_FACE('',(#856),#5900,.F.);
#6272=ADVANCED_FACE('',(#857),#5901,.F.);
#6273=ADVANCED_FACE('',(#858),#5902,.T.);
#6274=ADVANCED_FACE('',(#859),#5903,.T.);
#6275=ADVANCED_FACE('',(#860,#359,#360,#361,#362,#363),#329,.T.);
#6276=ADVANCED_FACE('',(#861,#364,#365,#366,#367,#368),#330,.F.);
#6277=ADVANCED_FACE('',(#862),#331,.F.);
#6278=ADVANCED_FACE('',(#863),#5904,.T.);
#6279=ADVANCED_FACE('',(#864),#5905,.T.);
#6280=ADVANCED_FACE('',(#865),#332,.F.);
#6281=ADVANCED_FACE('',(#866),#333,.F.);
#6282=ADVANCED_FACE('',(#867),#5906,.F.);
#6283=ADVANCED_FACE('',(#868),#334,.F.);
#6284=ADVANCED_FACE('',(#869),#494,.T.);
#6285=ADVANCED_FACE('',(#870),#5907,.T.);
#6286=ADVANCED_FACE('',(#871),#5908,.T.);
#6287=ADVANCED_FACE('',(#872),#495,.T.);
#6288=ADVANCED_FACE('',(#873),#496,.T.);
#6289=ADVANCED_FACE('',(#874),#5909,.T.);
#6290=ADVANCED_FACE('',(#875),#5910,.T.);
#6291=ADVANCED_FACE('',(#876),#497,.T.);
#6292=ADVANCED_FACE('',(#877),#5911,.T.);
#6293=ADVANCED_FACE('',(#878),#5912,.T.);
#6294=ADVANCED_FACE('',(#879),#498,.T.);
#6295=ADVANCED_FACE('',(#880),#499,.T.);
#6296=ADVANCED_FACE('',(#881),#5913,.T.);
#6297=ADVANCED_FACE('',(#882),#5914,.T.);
#6305=CLOSED_SHELL('',(#6254,#6255,#6256,#6257,#6258,#6259,#6260,#6261,
#6262,#6263,#6264,#6265,#6266,#6267,#6268,#6269,#6270,#6271,#6272,#6273,
#6274,#6275,#6276,#6277,#6278,#6279,#6280,#6281,#6282,#6283,#6284,#6285,
#6286,#6287,#6288,#6289,#6290,#6291,#6292,#6293,#6294,#6295,#6296,#6297));
#7055=AXIS2_PLACEMENT_3D('',#40531,#8783,#8784);
#7056=AXIS2_PLACEMENT_3D('',#40532,#8785,#8786);
#7057=AXIS2_PLACEMENT_3D('',#40535,#8787,#8788);
#7058=AXIS2_PLACEMENT_3D('',#40552,#8789,#8790);
#7059=AXIS2_PLACEMENT_3D('',#40553,#8791,#8792);
#7060=AXIS2_PLACEMENT_3D('',#40554,#8793,#8794);
#7061=AXIS2_PLACEMENT_3D('',#40557,#8795,#8796);
#7062=AXIS2_PLACEMENT_3D('',#40559,#8797,#8798);
#7063=AXIS2_PLACEMENT_3D('',#40561,#8799,#8800);
#7064=AXIS2_PLACEMENT_3D('',#40562,#8801,#8802);
#7065=AXIS2_PLACEMENT_3D('',#40563,#8803,#8804);
#7066=AXIS2_PLACEMENT_3D('',#40566,#8805,#8806);
#7067=AXIS2_PLACEMENT_3D('',#40583,#8807,#8808);
#7068=AXIS2_PLACEMENT_3D('',#40584,#8809,#8810);
#7069=AXIS2_PLACEMENT_3D('',#40585,#8811,#8812);
#7070=AXIS2_PLACEMENT_3D('',#40588,#8813,#8814);
#7071=AXIS2_PLACEMENT_3D('',#40590,#8815,#8816);
#7072=AXIS2_PLACEMENT_3D('',#40592,#8817,#8818);
#7073=AXIS2_PLACEMENT_3D('',#40593,#8819,#8820);
#7074=AXIS2_PLACEMENT_3D('',#40594,#8821,#8822);
#7075=AXIS2_PLACEMENT_3D('',#40597,#8823,#8824);
#7076=AXIS2_PLACEMENT_3D('',#40598,#8825,#8826);
#7077=AXIS2_PLACEMENT_3D('',#40601,#8828,#8829);
#7078=AXIS2_PLACEMENT_3D('',#40602,#8830,#8831);
#7079=AXIS2_PLACEMENT_3D('',#40604,#8832,#8833);
#7080=AXIS2_PLACEMENT_3D('',#40607,#8835,#8836);
#7081=AXIS2_PLACEMENT_3D('',#40608,#8837,#8838);
#7082=AXIS2_PLACEMENT_3D('',#40611,#8839,#8840);
#7083=AXIS2_PLACEMENT_3D('',#40612,#8841,#8842);
#7084=AXIS2_PLACEMENT_3D('',#40615,#8844,#8845);
#7085=AXIS2_PLACEMENT_3D('',#40616,#8846,#8847);
#7086=AXIS2_PLACEMENT_3D('',#40618,#8848,#8849);
#7087=AXIS2_PLACEMENT_3D('',#40621,#8851,#8852);
#7088=AXIS2_PLACEMENT_3D('',#40622,#8853,#8854);
#7089=AXIS2_PLACEMENT_3D('',#40625,#8855,#8856);
#7090=AXIS2_PLACEMENT_3D('',#40626,#8857,#8858);
#7091=AXIS2_PLACEMENT_3D('',#40629,#8860,#8861);
#7092=AXIS2_PLACEMENT_3D('',#40630,#8862,#8863);
#7093=AXIS2_PLACEMENT_3D('',#40632,#8864,#8865);
#7094=AXIS2_PLACEMENT_3D('',#40635,#8867,#8868);
#7095=AXIS2_PLACEMENT_3D('',#40636,#8869,#8870);
#7096=AXIS2_PLACEMENT_3D('',#40639,#8871,#8872);
#7097=AXIS2_PLACEMENT_3D('',#40640,#8873,#8874);
#7098=AXIS2_PLACEMENT_3D('',#40643,#8876,#8877);
#7099=AXIS2_PLACEMENT_3D('',#40644,#8878,#8879);
#7100=AXIS2_PLACEMENT_3D('',#40646,#8880,#8881);
#7101=AXIS2_PLACEMENT_3D('',#40649,#8883,#8884);
#7102=AXIS2_PLACEMENT_3D('',#40650,#8885,#8886);
#7103=AXIS2_PLACEMENT_3D('',#40653,#8887,#8888);
#7104=AXIS2_PLACEMENT_3D('',#40654,#8889,#8890);
#7105=AXIS2_PLACEMENT_3D('',#40657,#8892,#8893);
#7106=AXIS2_PLACEMENT_3D('',#40658,#8894,#8895);
#7107=AXIS2_PLACEMENT_3D('',#40660,#8896,#8897);
#7108=AXIS2_PLACEMENT_3D('',#40663,#8899,#8900);
#7109=AXIS2_PLACEMENT_3D('',#40664,#8901,#8902);
#7110=AXIS2_PLACEMENT_3D('',#40666,#8904,#8905);
#7111=AXIS2_PLACEMENT_3D('',#40668,#8907,#8908);
#7112=AXIS2_PLACEMENT_3D('',#40670,#8910,#8911);
#7113=AXIS2_PLACEMENT_3D('',#40672,#8913,#8914);
#7114=AXIS2_PLACEMENT_3D('',#40674,#8916,#8917);
#7115=AXIS2_PLACEMENT_3D('',#40677,#8918,#8919);
#7116=AXIS2_PLACEMENT_3D('',#40681,#8921,#8922);
#7117=AXIS2_PLACEMENT_3D('',#40683,#8924,#8925);
#7118=AXIS2_PLACEMENT_3D('',#40686,#8926,#8927);
#7119=AXIS2_PLACEMENT_3D('',#40690,#8929,#8930);
#7120=AXIS2_PLACEMENT_3D('',#40692,#8932,#8933);
#7121=AXIS2_PLACEMENT_3D('',#40698,#8936,#8937);
#7122=AXIS2_PLACEMENT_3D('',#40701,#8939,#8940);
#7123=AXIS2_PLACEMENT_3D('',#40704,#8942,#8943);
#7124=AXIS2_PLACEMENT_3D('',#40705,#8944,#8945);
#7125=AXIS2_PLACEMENT_3D('',#40711,#8948,#8949);
#7126=AXIS2_PLACEMENT_3D('',#40714,#8951,#8952);
#7127=AXIS2_PLACEMENT_3D('',#40717,#8954,#8955);
#7128=AXIS2_PLACEMENT_3D('',#40718,#8956,#8957);
#7129=AXIS2_PLACEMENT_3D('',#40722,#8961,#8962);
#7130=AXIS2_PLACEMENT_3D('',#40724,#8964,#8965);
#7131=AXIS2_PLACEMENT_3D('',#40726,#8966,#8967);
#7132=AXIS2_PLACEMENT_3D('',#40729,#8969,#8970);
#7133=AXIS2_PLACEMENT_3D('',#40730,#8971,#8972);
#7134=AXIS2_PLACEMENT_3D('',#40733,#8975,#8976);
#7135=AXIS2_PLACEMENT_3D('',#40737,#8980,#8981);
#7136=AXIS2_PLACEMENT_3D('',#40739,#8983,#8984);
#7137=AXIS2_PLACEMENT_3D('',#40742,#8987,#8988);
#7138=AXIS2_PLACEMENT_3D('',#40743,#8989,#8990);
#7139=AXIS2_PLACEMENT_3D('',#40744,#8991,#8992);
#7140=AXIS2_PLACEMENT_3D('',#40745,#8993,#8994);
#7141=AXIS2_PLACEMENT_3D('',#40746,#8995,#8996);
#7142=AXIS2_PLACEMENT_3D('',#40747,#8997,#8998);
#7143=AXIS2_PLACEMENT_3D('',#40748,#8999,#9000);
#7144=AXIS2_PLACEMENT_3D('',#40749,#9001,#9002);
#7145=AXIS2_PLACEMENT_3D('',#40750,#9003,#9004);
#7146=AXIS2_PLACEMENT_3D('',#40751,#9005,#9006);
#7147=AXIS2_PLACEMENT_3D('',#40752,#9007,#9008);
#7148=AXIS2_PLACEMENT_3D('',#40753,#9009,#9010);
#7149=AXIS2_PLACEMENT_3D('',#40754,#9011,#9012);
#7150=AXIS2_PLACEMENT_3D('',#40755,#9013,#9014);
#7151=AXIS2_PLACEMENT_3D('',#40756,#9015,#9016);
#7152=AXIS2_PLACEMENT_3D('',#40757,#9017,#9018);
#7153=AXIS2_PLACEMENT_3D('',#40758,#9019,#9020);
#7154=AXIS2_PLACEMENT_3D('',#40759,#9021,#9022);
#7155=AXIS2_PLACEMENT_3D('',#40760,#9023,#9024);
#7156=AXIS2_PLACEMENT_3D('',#40761,#9025,#9026);
#7157=AXIS2_PLACEMENT_3D('',#40762,#9027,#9028);
#7158=AXIS2_PLACEMENT_3D('',#40763,#9029,#9030);
#7159=AXIS2_PLACEMENT_3D('',#40764,#9031,#9032);
#7160=AXIS2_PLACEMENT_3D('',#40765,#9033,#9034);
#8783=DIRECTION('axis',(0.,0.,1.));
#8784=DIRECTION('refdir',(1.,0.,0.));
#8785=DIRECTION('center_axis',(0.,0.,1.));
#8786=DIRECTION('ref_axis',(1.,0.,0.));
#8787=DIRECTION('center_axis',(0.,0.,-1.));
#8788=DIRECTION('ref_axis',(1.,0.,0.));
#8789=DIRECTION('center_axis',(0.,0.,1.));
#8790=DIRECTION('ref_axis',(1.,0.,0.));
#8791=DIRECTION('center_axis',(1.,0.,0.));
#8792=DIRECTION('ref_axis',(0.,0.,-1.));
#8793=DIRECTION('center_axis',(0.,0.,1.));
#8794=DIRECTION('ref_axis',(1.,0.,0.));
#8795=DIRECTION('center_axis',(0.,0.,-1.));
#8796=DIRECTION('ref_axis',(1.,0.,0.));
#8797=DIRECTION('center_axis',(0.406935888454085,-0.913456721847338,0.));
#8798=DIRECTION('ref_axis',(0.913456721847338,0.406935888454085,0.));
#8799=DIRECTION('center_axis',(0.,0.,1.));
#8800=DIRECTION('ref_axis',(1.,0.,0.));
#8801=DIRECTION('center_axis',(-1.,0.,0.));
#8802=DIRECTION('ref_axis',(0.,0.,1.));
#8803=DIRECTION('center_axis',(0.,0.,1.));
#8804=DIRECTION('ref_axis',(1.,0.,0.));
#8805=DIRECTION('center_axis',(0.,0.,-1.));
#8806=DIRECTION('ref_axis',(1.,0.,0.));
#8807=DIRECTION('center_axis',(0.,0.,1.));
#8808=DIRECTION('ref_axis',(1.,0.,0.));
#8809=DIRECTION('center_axis',(1.,0.,0.));
#8810=DIRECTION('ref_axis',(0.,0.,-1.));
#8811=DIRECTION('center_axis',(0.,0.,1.));
#8812=DIRECTION('ref_axis',(1.,0.,0.));
#8813=DIRECTION('center_axis',(0.,0.,-1.));
#8814=DIRECTION('ref_axis',(1.,0.,0.));
#8815=DIRECTION('center_axis',(0.406935888454085,-0.913456721847338,0.));
#8816=DIRECTION('ref_axis',(0.913456721847338,0.406935888454085,0.));
#8817=DIRECTION('center_axis',(0.,0.,1.));
#8818=DIRECTION('ref_axis',(1.,0.,0.));
#8819=DIRECTION('center_axis',(-1.,0.,0.));
#8820=DIRECTION('ref_axis',(0.,0.,1.));
#8821=DIRECTION('center_axis',(0.,0.,1.));
#8822=DIRECTION('ref_axis',(1.,0.,0.));
#8823=DIRECTION('center_axis',(0.,0.,1.));
#8824=DIRECTION('ref_axis',(1.,0.,0.));
#8825=DIRECTION('center_axis',(0.,0.,1.));
#8826=DIRECTION('ref_axis',(1.,0.,0.));
#8827=DIRECTION('',(-0.707106781186539,-8.65956056235483E-17,0.707106781186556));
#8828=DIRECTION('center_axis',(0.,0.,-1.));
#8829=DIRECTION('ref_axis',(1.,0.,0.));
#8830=DIRECTION('center_axis',(0.,0.,-1.));
#8831=DIRECTION('ref_axis',(-1.,0.,0.));
#8832=DIRECTION('center_axis',(0.,0.,-1.));
#8833=DIRECTION('ref_axis',(1.,0.,0.));
#8834=DIRECTION('',(0.707106781186516,-8.65956056235455E-17,-0.707106781186578));
#8835=DIRECTION('center_axis',(0.,0.,1.));
#8836=DIRECTION('ref_axis',(1.,0.,0.));
#8837=DIRECTION('center_axis',(0.,0.,1.));
#8838=DIRECTION('ref_axis',(1.,0.,0.));
#8839=DIRECTION('center_axis',(0.,0.,1.));
#8840=DIRECTION('ref_axis',(1.,0.,0.));
#8841=DIRECTION('center_axis',(0.,0.,1.));
#8842=DIRECTION('ref_axis',(1.,0.,0.));
#8843=DIRECTION('',(-0.707106781186539,-8.65956056235482E-17,0.707106781186556));
#8844=DIRECTION('center_axis',(0.,0.,-1.));
#8845=DIRECTION('ref_axis',(1.,0.,0.));
#8846=DIRECTION('center_axis',(0.,0.,-1.));
#8847=DIRECTION('ref_axis',(-1.,0.,0.));
#8848=DIRECTION('center_axis',(0.,0.,-1.));
#8849=DIRECTION('ref_axis',(1.,0.,0.));
#8850=DIRECTION('',(0.707106781186533,-8.65956056235476E-17,-0.707106781186561));
#8851=DIRECTION('center_axis',(0.,0.,1.));
#8852=DIRECTION('ref_axis',(1.,0.,0.));
#8853=DIRECTION('center_axis',(0.,0.,1.));
#8854=DIRECTION('ref_axis',(1.,0.,0.));
#8855=DIRECTION('center_axis',(0.,0.,1.));
#8856=DIRECTION('ref_axis',(1.,0.,0.));
#8857=DIRECTION('center_axis',(0.,0.,1.));
#8858=DIRECTION('ref_axis',(1.,0.,0.));
#8859=DIRECTION('',(-0.707106781186539,-8.65956056235482E-17,0.707106781186556));
#8860=DIRECTION('center_axis',(0.,0.,-1.));
#8861=DIRECTION('ref_axis',(1.,0.,0.));
#8862=DIRECTION('center_axis',(0.,0.,-1.));
#8863=DIRECTION('ref_axis',(-1.,0.,0.));
#8864=DIRECTION('center_axis',(0.,0.,-1.));
#8865=DIRECTION('ref_axis',(1.,0.,0.));
#8866=DIRECTION('',(0.707106781186539,-8.65956056235483E-17,-0.707106781186556));
#8867=DIRECTION('center_axis',(0.,0.,1.));
#8868=DIRECTION('ref_axis',(1.,0.,0.));
#8869=DIRECTION('center_axis',(0.,0.,1.));
#8870=DIRECTION('ref_axis',(1.,0.,0.));
#8871=DIRECTION('center_axis',(0.,0.,1.));
#8872=DIRECTION('ref_axis',(1.,0.,0.));
#8873=DIRECTION('center_axis',(0.,0.,1.));
#8874=DIRECTION('ref_axis',(1.,0.,0.));
#8875=DIRECTION('',(-0.707106781186538,-8.65956056235482E-17,0.707106781186557));
#8876=DIRECTION('center_axis',(0.,0.,-1.));
#8877=DIRECTION('ref_axis',(1.,0.,0.));
#8878=DIRECTION('center_axis',(0.,0.,-1.));
#8879=DIRECTION('ref_axis',(-1.,0.,0.));
#8880=DIRECTION('center_axis',(0.,0.,-1.));
#8881=DIRECTION('ref_axis',(1.,0.,0.));
#8882=DIRECTION('',(0.707106781186538,-8.65956056235482E-17,-0.707106781186557));
#8883=DIRECTION('center_axis',(0.,0.,1.));
#8884=DIRECTION('ref_axis',(1.,0.,0.));
#8885=DIRECTION('center_axis',(0.,0.,1.));
#8886=DIRECTION('ref_axis',(1.,0.,0.));
#8887=DIRECTION('center_axis',(0.,0.,1.));
#8888=DIRECTION('ref_axis',(1.,0.,0.));
#8889=DIRECTION('center_axis',(0.,0.,1.));
#8890=DIRECTION('ref_axis',(1.,0.,0.));
#8891=DIRECTION('',(-0.707106781186538,-8.65956056235482E-17,0.707106781186557));
#8892=DIRECTION('center_axis',(0.,0.,-1.));
#8893=DIRECTION('ref_axis',(1.,0.,0.));
#8894=DIRECTION('center_axis',(0.,0.,-1.));
#8895=DIRECTION('ref_axis',(-1.,0.,0.));
#8896=DIRECTION('center_axis',(0.,0.,-1.));
#8897=DIRECTION('ref_axis',(1.,0.,0.));
#8898=DIRECTION('',(0.707106781186558,-8.65956056235506E-17,-0.707106781186537));
#8899=DIRECTION('center_axis',(0.,0.,1.));
#8900=DIRECTION('ref_axis',(1.,0.,0.));
#8901=DIRECTION('center_axis',(0.,0.,-1.));
#8902=DIRECTION('ref_axis',(-1.,0.,0.));
#8903=DIRECTION('',(0.,0.,-1.));
#8904=DIRECTION('center_axis',(0.,0.,-1.));
#8905=DIRECTION('ref_axis',(-1.,0.,0.));
#8906=DIRECTION('',(0.,0.,-1.));
#8907=DIRECTION('center_axis',(0.,0.,-1.));
#8908=DIRECTION('ref_axis',(-1.,0.,0.));
#8909=DIRECTION('',(0.,0.,-1.));
#8910=DIRECTION('center_axis',(0.,0.,-1.));
#8911=DIRECTION('ref_axis',(-1.,0.,0.));
#8912=DIRECTION('',(0.,0.,-1.));
#8913=DIRECTION('center_axis',(0.,0.,-1.));
#8914=DIRECTION('ref_axis',(-1.,0.,0.));
#8915=DIRECTION('',(0.,0.,-1.));
#8916=DIRECTION('center_axis',(0.,0.,-1.));
#8917=DIRECTION('ref_axis',(-1.,0.,0.));
#8918=DIRECTION('center_axis',(0.,0.,-1.));
#8919=DIRECTION('ref_axis',(1.,1.04083408558608E-14,0.));
#8920=DIRECTION('',(0.,0.,-1.));
#8921=DIRECTION('center_axis',(0.,0.,1.));
#8922=DIRECTION('ref_axis',(1.,0.,0.));
#8923=DIRECTION('',(0.,0.,-1.));
#8924=DIRECTION('center_axis',(0.,0.,-1.));
#8925=DIRECTION('ref_axis',(-1.,0.,0.));
#8926=DIRECTION('center_axis',(0.,0.,-1.));
#8927=DIRECTION('ref_axis',(1.,0.,0.));
#8928=DIRECTION('',(0.,0.,-1.));
#8929=DIRECTION('center_axis',(0.,0.,1.));
#8930=DIRECTION('ref_axis',(1.,0.,0.));
#8931=DIRECTION('',(0.,0.,-1.));
#8932=DIRECTION('center_axis',(0.,0.,1.));
#8933=DIRECTION('ref_axis',(1.,0.,0.));
#8934=DIRECTION('',(0.370256409888397,-0.928929594176305,0.));
#8935=DIRECTION('',(-1.,-1.28820497806328E-16,0.));
#8936=DIRECTION('center_axis',(0.,0.,1.));
#8937=DIRECTION('ref_axis',(1.,0.,0.));
#8938=DIRECTION('',(1.,-8.88417226250542E-18,0.));
#8939=DIRECTION('center_axis',(0.,0.,1.));
#8940=DIRECTION('ref_axis',(1.,0.,0.));
#8941=DIRECTION('',(-0.866025403784438,-0.500000000000001,0.));
#8942=DIRECTION('center_axis',(0.,0.,1.));
#8943=DIRECTION('ref_axis',(1.,0.,0.));
#8944=DIRECTION('center_axis',(0.,0.,1.));
#8945=DIRECTION('ref_axis',(1.,0.,0.));
#8946=DIRECTION('',(1.,1.28820497806328E-16,0.));
#8947=DIRECTION('',(-0.370256409888397,0.928929594176305,0.));
#8948=DIRECTION('center_axis',(0.,0.,-1.));
#8949=DIRECTION('ref_axis',(1.,4.16333634234433E-15,0.));
#8950=DIRECTION('',(0.866025403784438,0.500000000000001,0.));
#8951=DIRECTION('center_axis',(0.,0.,-1.));
#8952=DIRECTION('ref_axis',(1.,0.,0.));
#8953=DIRECTION('',(-1.,8.88417226250542E-18,0.));
#8954=DIRECTION('center_axis',(0.,0.,-1.));
#8955=DIRECTION('ref_axis',(1.,0.,0.));
#8956=DIRECTION('center_axis',(8.88417226250541E-18,1.,0.));
#8957=DIRECTION('ref_axis',(-1.,8.88417226250541E-18,0.));
#8958=DIRECTION('',(0.,0.,-1.));
#8959=DIRECTION('',(-1.,8.88417226250542E-18,0.));
#8960=DIRECTION('',(1.,-8.88417226250542E-18,0.));
#8961=DIRECTION('center_axis',(0.,0.,-1.));
#8962=DIRECTION('ref_axis',(0.838729959061342,-0.544547569798048,0.));
#8963=DIRECTION('',(0.,0.,-1.));
#8964=DIRECTION('center_axis',(0.,0.,-1.));
#8965=DIRECTION('ref_axis',(-1.,0.,0.));
#8966=DIRECTION('center_axis',(0.,0.,1.));
#8967=DIRECTION('ref_axis',(1.,0.,0.));
#8968=DIRECTION('',(0.,0.,-1.));
#8969=DIRECTION('center_axis',(0.,0.,-1.));
#8970=DIRECTION('ref_axis',(1.,-2.31296463463574E-15,0.));
#8971=DIRECTION('center_axis',(0.500000000000001,-0.866025403784438,0.));
#8972=DIRECTION('ref_axis',(0.866025403784438,0.500000000000001,0.));
#8973=DIRECTION('',(-0.866025403784438,-0.500000000000001,0.));
#8974=DIRECTION('',(0.866025403784438,0.500000000000001,0.));
#8975=DIRECTION('center_axis',(0.928929594176305,0.370256409888397,0.));
#8976=DIRECTION('ref_axis',(-0.370256409888397,0.928929594176305,0.));
#8977=DIRECTION('',(0.370256409888397,-0.928929594176305,0.));
#8978=DIRECTION('',(0.,0.,-1.));
#8979=DIRECTION('',(-0.370256409888397,0.928929594176305,0.));
#8980=DIRECTION('center_axis',(0.,0.,-1.));
#8981=DIRECTION('ref_axis',(0.712771275806866,-0.701396541468984,0.));
#8982=DIRECTION('',(0.,0.,-1.));
#8983=DIRECTION('center_axis',(1.28820497806328E-16,-1.,0.));
#8984=DIRECTION('ref_axis',(1.,1.28820497806328E-16,0.));
#8985=DIRECTION('',(-1.,-1.28820497806328E-16,0.));
#8986=DIRECTION('',(1.,1.28820497806328E-16,0.));
#8987=DIRECTION('center_axis',(0.,0.,1.));
#8988=DIRECTION('ref_axis',(1.,0.,0.));
#8989=DIRECTION('center_axis',(-0.866025403784439,-0.499999999999999,0.));
#8990=DIRECTION('ref_axis',(0.499999999999999,-0.86602540378444,0.));
#8991=DIRECTION('center_axis',(-0.866025403784438,-0.500000000000001,0.));
#8992=DIRECTION('ref_axis',(0.500000000000001,-0.866025403784438,0.));
#8993=DIRECTION('center_axis',(-0.866025403784439,-0.499999999999999,0.));
#8994=DIRECTION('ref_axis',(0.499999999999999,-0.86602540378444,0.));
#8995=DIRECTION('center_axis',(1.,-8.88417226250541E-18,0.));
#8996=DIRECTION('ref_axis',(8.88417226250541E-18,1.,0.));
#8997=DIRECTION('center_axis',(-1.,0.,0.));
#8998=DIRECTION('ref_axis',(0.,0.,1.));
#8999=DIRECTION('center_axis',(0.,0.,1.));
#9000=DIRECTION('ref_axis',(-0.944752944945269,0.327783271411525,0.));
#9001=DIRECTION('center_axis',(0.370256409888406,-0.928929594176302,0.));
#9002=DIRECTION('ref_axis',(0.928929594176302,0.370256409888406,0.));
#9003=DIRECTION('center_axis',(0.,0.,1.));
#9004=DIRECTION('ref_axis',(-1.,-1.18852590797403E-16,0.));
#9005=DIRECTION('center_axis',(1.,0.,0.));
#9006=DIRECTION('ref_axis',(0.,0.,-1.));
#9007=DIRECTION('center_axis',(0.370256409888397,-0.928929594176305,0.));
#9008=DIRECTION('ref_axis',(0.928929594176305,0.370256409888397,0.));
#9009=DIRECTION('center_axis',(-1.,-1.28820497806328E-16,0.));
#9010=DIRECTION('ref_axis',(1.28820497806329E-16,-1.,0.));
#9011=DIRECTION('center_axis',(0.,0.,1.));
#9012=DIRECTION('ref_axis',(1.,0.,0.));
#9013=DIRECTION('center_axis',(-0.866025403784439,-0.499999999999999,0.));
#9014=DIRECTION('ref_axis',(0.499999999999999,-0.86602540378444,0.));
#9015=DIRECTION('center_axis',(0.866025403784438,0.500000000000001,0.));
#9016=DIRECTION('ref_axis',(-0.500000000000001,0.866025403784438,0.));
#9017=DIRECTION('center_axis',(-0.866025403784443,-0.499999999999993,0.));
#9018=DIRECTION('ref_axis',(0.499999999999993,-0.866025403784443,0.));
#9019=DIRECTION('center_axis',(-1.,8.88417226250541E-18,0.));
#9020=DIRECTION('ref_axis',(-8.88417226250541E-18,-1.,0.));
#9021=DIRECTION('center_axis',(-1.,0.,0.));
#9022=DIRECTION('ref_axis',(0.,0.,1.));
#9023=DIRECTION('center_axis',(0.,0.,1.));
#9024=DIRECTION('ref_axis',(-0.944752944945269,0.327783271411525,0.));
#9025=DIRECTION('center_axis',(0.3702564098884,-0.928929594176304,0.));
#9026=DIRECTION('ref_axis',(0.928929594176304,0.3702564098884,0.));
#9027=DIRECTION('center_axis',(0.,0.,1.));
#9028=DIRECTION('ref_axis',(-1.,-1.18852590797403E-16,0.));
#9029=DIRECTION('center_axis',(1.,0.,0.));
#9030=DIRECTION('ref_axis',(0.,0.,-1.));
#9031=DIRECTION('center_axis',(-0.370256409888397,0.928929594176305,0.));
#9032=DIRECTION('ref_axis',(-0.928929594176305,-0.370256409888397,0.));
#9033=DIRECTION('center_axis',(1.,1.28820497806328E-16,0.));
#9034=DIRECTION('ref_axis',(-1.28820497806328E-16,1.,0.));
#40531=CARTESIAN_POINT('',(0.,0.,0.));
#40532=CARTESIAN_POINT('Origin',(152.4,23.371783782548,7.5));
#40533=CARTESIAN_POINT('',(168.776131634213,23.7277510548322,8.));
#40534=CARTESIAN_POINT('',(152.4,6.99178378254796,8.));
#40535=CARTESIAN_POINT('Origin',(152.4,23.371783782548,8.));
#40536=CARTESIAN_POINT('',(168.27794537285,23.6272260202514,7.5));
#40537=CARTESIAN_POINT('Ctrl Pts',(168.776131634213,23.7277510548321,8.));
#40538=CARTESIAN_POINT('Ctrl Pts',(168.775078472326,23.727537009893,8.));
#40539=CARTESIAN_POINT('Ctrl Pts',(168.774025310872,23.7273229746447,7.99999664467033));
#40540=CARTESIAN_POINT('Ctrl Pts',(168.707149864385,23.7137324075318,7.99957051796987));
#40541=CARTESIAN_POINT('Ctrl Pts',(168.641973161379,23.7005259564475,7.98604806346216));
#40542=CARTESIAN_POINT('Ctrl Pts',(168.521018609496,23.6760802664691,7.93442027877329));
#40543=CARTESIAN_POINT('Ctrl Pts',(168.466249273604,23.6650436658758,7.89698073370765));
#40544=CARTESIAN_POINT('Ctrl Pts',(168.374932604161,23.6466749169578,7.80338879792307));
#40545=CARTESIAN_POINT('Ctrl Pts',(168.338969416124,23.6394586601229,7.74845769049294));
#40546=CARTESIAN_POINT('Ctrl Pts',(168.290420014211,23.629723437839,7.6284017905508));
#40547=CARTESIAN_POINT('Ctrl Pts',(168.277978201841,23.6272325959581,7.56467314065448));
#40548=CARTESIAN_POINT('Ctrl Pts',(168.277945394473,23.6272260245827,7.50017006215143));
#40549=CARTESIAN_POINT('Ctrl Pts',(168.27794537285,23.6272260202515,7.5000850304854));
#40550=CARTESIAN_POINT('Ctrl Pts',(168.27794537285,23.6272260202515,7.5));
#40551=CARTESIAN_POINT('',(152.4,7.49178378254796,7.5));
#40552=CARTESIAN_POINT('Origin',(152.4,23.371783782548,7.5));
#40553=CARTESIAN_POINT('Origin',(152.4,6.99178378254796,7.5));
#40554=CARTESIAN_POINT('Origin',(152.4,23.371783782548,7.5));
#40555=CARTESIAN_POINT('',(181.411385485872,36.2960675998495,7.5));
#40556=CARTESIAN_POINT('',(152.4,-8.38821621745206,7.5));
#40557=CARTESIAN_POINT('Origin',(152.4,23.371783782548,7.5));
#40558=CARTESIAN_POINT('',(180.954657124948,36.0925996556225,8.));
#40559=CARTESIAN_POINT('Origin',(180.954657124948,36.0925996556225,7.5));
#40560=CARTESIAN_POINT('',(152.4,-7.88821621745207,8.));
#40561=CARTESIAN_POINT('Origin',(152.4,23.371783782548,8.));
#40562=CARTESIAN_POINT('Origin',(152.4,-7.88821621745206,7.5));
#40563=CARTESIAN_POINT('Origin',(152.4,23.371783782548,-7.5));
#40564=CARTESIAN_POINT('',(168.27794537285,23.6272260202514,-7.5));
#40565=CARTESIAN_POINT('',(152.4,7.49178378254796,-7.5));
#40566=CARTESIAN_POINT('Origin',(152.4,23.371783782548,-7.5));
#40567=CARTESIAN_POINT('',(168.776131634213,23.7277510548321,-8.));
#40568=CARTESIAN_POINT('Ctrl Pts',(168.27794537285,23.6272260202514,-7.5));
#40569=CARTESIAN_POINT('Ctrl Pts',(168.27794537285,23.6272260202514,-7.50008503046509));
#40570=CARTESIAN_POINT('Ctrl Pts',(168.277945394473,23.6272260245825,-7.5001700621108));
#40571=CARTESIAN_POINT('Ctrl Pts',(168.277978201833,23.6272325959564,-7.56467314059333));
#40572=CARTESIAN_POINT('Ctrl Pts',(168.290420014195,23.6297234378358,-7.62840179049102));
#40573=CARTESIAN_POINT('Ctrl Pts',(168.338969416094,23.6394586601167,-7.74845769043869));
#40574=CARTESIAN_POINT('Ctrl Pts',(168.374932604124,23.6466749169502,-7.80338879787307));
#40575=CARTESIAN_POINT('Ctrl Pts',(168.466249273555,23.6650436658658,-7.89698073366876));
#40576=CARTESIAN_POINT('Ctrl Pts',(168.521018609442,23.6760802664581,-7.93442027874115));
#40577=CARTESIAN_POINT('Ctrl Pts',(168.641973161336,23.7005259564387,-7.98604806345277));
#40578=CARTESIAN_POINT('Ctrl Pts',(168.70714986435,23.7137324075447,-7.99957051796967));
#40579=CARTESIAN_POINT('Ctrl Pts',(168.774025310873,23.7273229746435,-7.99999664467033));
#40580=CARTESIAN_POINT('Ctrl Pts',(168.775078472325,23.7275370098928,-8.));
#40581=CARTESIAN_POINT('Ctrl Pts',(168.776131634213,23.727751054832,-8.));
#40582=CARTESIAN_POINT('',(152.4,6.99178378254796,-8.));
#40583=CARTESIAN_POINT('Origin',(152.4,23.371783782548,-8.));
#40584=CARTESIAN_POINT('Origin',(152.4,6.99178378254796,-7.5));
#40585=CARTESIAN_POINT('Origin',(152.4,23.371783782548,-7.5));
#40586=CARTESIAN_POINT('',(180.954657124948,36.0925996556225,-8.));
#40587=CARTESIAN_POINT('',(152.4,-7.88821621745207,-8.));
#40588=CARTESIAN_POINT('Origin',(152.4,23.371783782548,-8.));
#40589=CARTESIAN_POINT('',(181.411385485872,36.2960675998495,-7.5));
#40590=CARTESIAN_POINT('Origin',(180.954657124948,36.0925996556225,-7.5));
#40591=CARTESIAN_POINT('',(152.4,-8.38821621745206,-7.5));
#40592=CARTESIAN_POINT('Origin',(152.4,23.371783782548,-7.5));
#40593=CARTESIAN_POINT('Origin',(152.4,-7.88821621745206,-7.5));
#40594=CARTESIAN_POINT('Origin',(0.,0.,7.49999999999996));
#40595=CARTESIAN_POINT('',(3.5,4.28626379701574E-16,7.49999999999996));
#40596=CARTESIAN_POINT('',(-3.5,-4.28626379701574E-16,7.49999999999996));
#40597=CARTESIAN_POINT('Origin',(0.,0.,7.49999999999996));
#40598=CARTESIAN_POINT('Origin',(0.,0.,7.49999999999996));
#40599=CARTESIAN_POINT('',(-4.00000000000003,-4.89858719658945E-16,8.));
#40600=CARTESIAN_POINT('',(-3.5,-4.28626379701574E-16,7.49999999999996));
#40601=CARTESIAN_POINT('Origin',(0.,0.,8.));
#40602=CARTESIAN_POINT('Origin',(0.,0.,-8.));
#40603=CARTESIAN_POINT('',(3.5,-4.28626379701574E-16,-7.49999999999998));
#40604=CARTESIAN_POINT('Origin',(0.,0.,-7.49999999999998));
#40605=CARTESIAN_POINT('',(3.99999999999998,-4.89858719658938E-16,-8.));
#40606=CARTESIAN_POINT('',(3.99999999999998,-4.89858719658938E-16,-8.));
#40607=CARTESIAN_POINT('Origin',(0.,0.,-8.));
#40608=CARTESIAN_POINT('Origin',(25.4,0.,7.49999999999996));
#40609=CARTESIAN_POINT('',(28.9,4.28626379701574E-16,7.49999999999996));
#40610=CARTESIAN_POINT('',(21.9,-4.28626379701574E-16,7.49999999999996));
#40611=CARTESIAN_POINT('Origin',(25.4,0.,7.49999999999996));
#40612=CARTESIAN_POINT('Origin',(25.4,0.,7.49999999999996));
#40613=CARTESIAN_POINT('',(21.4,-4.89858719658945E-16,8.));
#40614=CARTESIAN_POINT('',(21.9,-4.28626379701574E-16,7.49999999999996));
#40615=CARTESIAN_POINT('Origin',(25.4,0.,8.));
#40616=CARTESIAN_POINT('Origin',(25.4,0.,-8.));
#40617=CARTESIAN_POINT('',(28.9,-4.28626379701574E-16,-7.49999999999998));
#40618=CARTESIAN_POINT('Origin',(25.4,0.,-7.49999999999998));
#40619=CARTESIAN_POINT('',(29.4,-4.89858719658942E-16,-8.));
#40620=CARTESIAN_POINT('',(29.4,-4.89858719658942E-16,-8.));
#40621=CARTESIAN_POINT('Origin',(25.4,0.,-8.));
#40622=CARTESIAN_POINT('Origin',(50.8,0.,7.49999999999996));
#40623=CARTESIAN_POINT('',(54.3,4.28626379701573E-16,7.49999999999996));
#40624=CARTESIAN_POINT('',(47.3,-4.28626379701574E-16,7.49999999999996));
#40625=CARTESIAN_POINT('Origin',(50.8,0.,7.49999999999996));
#40626=CARTESIAN_POINT('Origin',(50.8,0.,7.49999999999996));
#40627=CARTESIAN_POINT('',(46.8,-4.89858719658945E-16,8.));
#40628=CARTESIAN_POINT('',(47.3,-4.28626379701574E-16,7.49999999999996));
#40629=CARTESIAN_POINT('Origin',(50.8,0.,8.));
#40630=CARTESIAN_POINT('Origin',(50.8,0.,-8.));
#40631=CARTESIAN_POINT('',(54.3,-4.28626379701574E-16,-7.49999999999999));
#40632=CARTESIAN_POINT('Origin',(50.8,0.,-7.49999999999998));
#40633=CARTESIAN_POINT('',(54.8,-4.89858719658942E-16,-8.));
#40634=CARTESIAN_POINT('',(54.8,-4.89858719658942E-16,-8.));
#40635=CARTESIAN_POINT('Origin',(50.8,0.,-8.));
#40636=CARTESIAN_POINT('Origin',(76.2,0.,7.49999999999995));
#40637=CARTESIAN_POINT('',(79.7,4.28626379701573E-16,7.49999999999995));
#40638=CARTESIAN_POINT('',(72.7,-4.28626379701572E-16,7.49999999999995));
#40639=CARTESIAN_POINT('Origin',(76.2,0.,7.49999999999995));
#40640=CARTESIAN_POINT('Origin',(76.2,0.,7.49999999999995));
#40641=CARTESIAN_POINT('',(72.2,-4.89858719658946E-16,8.00000000000001));
#40642=CARTESIAN_POINT('',(72.7,-4.28626379701572E-16,7.49999999999995));
#40643=CARTESIAN_POINT('Origin',(76.2,0.,8.));
#40644=CARTESIAN_POINT('Origin',(76.2,0.,-8.));
#40645=CARTESIAN_POINT('',(79.7,-4.28626379701572E-16,-7.49999999999997));
#40646=CARTESIAN_POINT('Origin',(76.2,0.,-7.49999999999998));
#40647=CARTESIAN_POINT('',(80.2,-4.89858719658942E-16,-8.));
#40648=CARTESIAN_POINT('',(80.2,-4.89858719658942E-16,-8.));
#40649=CARTESIAN_POINT('Origin',(76.2,0.,-8.));
#40650=CARTESIAN_POINT('Origin',(101.6,0.,7.49999999999995));
#40651=CARTESIAN_POINT('',(105.1,4.28626379701573E-16,7.49999999999995));
#40652=CARTESIAN_POINT('',(98.1,-4.28626379701572E-16,7.49999999999995));
#40653=CARTESIAN_POINT('Origin',(101.6,0.,7.49999999999995));
#40654=CARTESIAN_POINT('Origin',(101.6,0.,7.49999999999995));
#40655=CARTESIAN_POINT('',(97.6,-4.89858719658945E-16,8.00000000000001));
#40656=CARTESIAN_POINT('',(98.1,-4.28626379701572E-16,7.49999999999995));
#40657=CARTESIAN_POINT('Origin',(101.6,0.,8.));
#40658=CARTESIAN_POINT('Origin',(101.6,0.,-8.));
#40659=CARTESIAN_POINT('',(105.1,-4.28626379701573E-16,-7.50000000000003));
#40660=CARTESIAN_POINT('Origin',(101.6,0.,-7.50000000000003));
#40661=CARTESIAN_POINT('',(105.6,-4.89858719658938E-16,-8.));
#40662=CARTESIAN_POINT('',(105.6,-4.89858719658938E-16,-8.));
#40663=CARTESIAN_POINT('Origin',(101.6,0.,-8.));
#40664=CARTESIAN_POINT('Origin',(101.6,0.,8.));
#40665=CARTESIAN_POINT('',(105.1,-4.28626379701572E-16,8.));
#40666=CARTESIAN_POINT('Origin',(76.2,0.,8.));
#40667=CARTESIAN_POINT('',(79.7,-4.28626379701572E-16,8.));
#40668=CARTESIAN_POINT('Origin',(50.8,0.,8.));
#40669=CARTESIAN_POINT('',(54.3,-4.28626379701574E-16,8.));
#40670=CARTESIAN_POINT('Origin',(25.4,0.,8.));
#40671=CARTESIAN_POINT('',(28.9,-4.28626379701574E-16,8.));
#40672=CARTESIAN_POINT('Origin',(0.,0.,8.));
#40673=CARTESIAN_POINT('',(3.5,-4.28626379701574E-16,8.));
#40674=CARTESIAN_POINT('Origin',(169.138185555828,29.5714781038137,8.));
#40675=CARTESIAN_POINT('',(166.351396773299,28.4607088741485,7.5));
#40676=CARTESIAN_POINT('',(167.638185555828,32.169554315167,7.5));
#40677=CARTESIAN_POINT('Origin',(169.138185555828,29.5714781038137,7.5));
#40678=CARTESIAN_POINT('',(167.638185555828,32.169554315167,-7.5));
#40679=CARTESIAN_POINT('',(167.638185555828,32.169554315167,8.));
#40680=CARTESIAN_POINT('',(166.351396773299,28.4607088741485,-7.5));
#40681=CARTESIAN_POINT('Origin',(169.138185555828,29.5714781038137,-7.5));
#40682=CARTESIAN_POINT('',(166.351396773299,28.4607088741485,8.));
#40683=CARTESIAN_POINT('Origin',(-42.86,-0.448216217452066,8.));
#40684=CARTESIAN_POINT('',(-42.86,-8.38821621745207,7.5));
#40685=CARTESIAN_POINT('',(-42.86,7.49178378254793,7.5));
#40686=CARTESIAN_POINT('Origin',(-42.86,-0.448216217452066,7.5));
#40687=CARTESIAN_POINT('',(-42.86,7.49178378254793,-7.5));
#40688=CARTESIAN_POINT('',(-42.86,7.49178378254793,8.));
#40689=CARTESIAN_POINT('',(-42.86,-8.38821621745207,-7.5));
#40690=CARTESIAN_POINT('Origin',(-42.86,-0.448216217452066,-7.5));
#40691=CARTESIAN_POINT('',(-42.86,-8.38821621745207,8.));
#40692=CARTESIAN_POINT('Origin',(-42.86,-0.448216217452066,8.));
#40693=CARTESIAN_POINT('',(166.815861570388,28.6458370790927,8.));
#40694=CARTESIAN_POINT('',(168.742410169938,23.8123542251956,8.));
#40695=CARTESIAN_POINT('',(-42.86,6.99178378254793,8.));
#40696=CARTESIAN_POINT('',(-42.86,6.99178378254793,8.));
#40697=CARTESIAN_POINT('',(-42.86,-7.88821621745207,8.));
#40698=CARTESIAN_POINT('Origin',(-42.86,-0.448216217452066,8.));
#40699=CARTESIAN_POINT('',(152.4,-7.88821621745207,8.));
#40700=CARTESIAN_POINT('',(177.42101532033,37.2403234439484,8.));
#40701=CARTESIAN_POINT('Origin',(178.67101532033,35.0752599344873,8.));
#40702=CARTESIAN_POINT('',(167.888185555828,31.7365416132748,8.));
#40703=CARTESIAN_POINT('',(167.888185555829,31.7365416132748,8.));
#40704=CARTESIAN_POINT('Origin',(169.138185555828,29.5714781038137,8.));
#40705=CARTESIAN_POINT('Origin',(-42.86,-0.448216217452066,-8.));
#40706=CARTESIAN_POINT('',(-42.86,6.99178378254793,-8.));
#40707=CARTESIAN_POINT('',(-42.86,6.99178378254793,-8.));
#40708=CARTESIAN_POINT('',(166.815861570388,28.6458370790927,-8.));
#40709=CARTESIAN_POINT('',(148.078108595041,75.6566458113737,-8.));
#40710=CARTESIAN_POINT('',(167.888185555828,31.7365416132748,-8.));
#40711=CARTESIAN_POINT('Origin',(169.138185555828,29.5714781038137,-8.));
#40712=CARTESIAN_POINT('',(177.42101532033,37.2403234439484,-8.));
#40713=CARTESIAN_POINT('',(-4.10936255907258,-67.5662890908191,-8.));
#40714=CARTESIAN_POINT('Origin',(178.67101532033,35.0752599344873,-8.));
#40715=CARTESIAN_POINT('',(-42.86,-7.88821621745207,-8.));
#40716=CARTESIAN_POINT('',(-42.86,-7.88821621745207,-8.));
#40717=CARTESIAN_POINT('Origin',(-42.86,-0.448216217452066,-8.));
#40718=CARTESIAN_POINT('Origin',(-42.86,-8.38821621745207,8.));
#40719=CARTESIAN_POINT('',(152.4,-8.38821621745206,8.));
#40720=CARTESIAN_POINT('',(-42.86,-8.38821621745207,7.5));
#40721=CARTESIAN_POINT('',(-42.86,-8.38821621745207,-7.5));
#40722=CARTESIAN_POINT('Origin',(152.4,23.371783782548,8.));
#40723=CARTESIAN_POINT('',(181.411385485872,36.2960675998495,8.));
#40724=CARTESIAN_POINT('Origin',(178.67101532033,35.0752599344873,8.));
#40725=CARTESIAN_POINT('',(177.17101532033,37.6733361458406,-7.5));
#40726=CARTESIAN_POINT('Origin',(178.67101532033,35.0752599344873,-7.5));
#40727=CARTESIAN_POINT('',(177.17101532033,37.6733361458406,7.5));
#40728=CARTESIAN_POINT('',(177.17101532033,37.6733361458406,8.));
#40729=CARTESIAN_POINT('Origin',(178.67101532033,35.0752599344873,7.5));
#40730=CARTESIAN_POINT('Origin',(167.638185555828,32.169554315167,8.));
#40731=CARTESIAN_POINT('',(167.638185555828,32.169554315167,-7.5));
#40732=CARTESIAN_POINT('',(177.17101532033,37.6733361458406,7.5));
#40733=CARTESIAN_POINT('Origin',(168.27794537285,23.6272260202514,8.));
#40734=CARTESIAN_POINT('',(168.27794537285,23.6272260202514,-7.5));
#40735=CARTESIAN_POINT('',(168.27794537285,23.6272260202514,8.));
#40736=CARTESIAN_POINT('',(166.351396773299,28.4607088741485,7.5));
#40737=CARTESIAN_POINT('Origin',(152.4,23.371783782548,8.));
#40738=CARTESIAN_POINT('',(152.4,7.49178378254796,8.));
#40739=CARTESIAN_POINT('Origin',(152.4,7.49178378254796,8.));
#40740=CARTESIAN_POINT('',(152.4,7.49178378254796,-7.5));
#40741=CARTESIAN_POINT('',(152.4,7.49178378254796,7.5));
#40742=CARTESIAN_POINT('Origin',(178.67101532033,35.0752599344873,-7.5));
#40743=CARTESIAN_POINT('Origin',(177.42101532033,37.2403234439484,-7.5));
#40744=CARTESIAN_POINT('Origin',(167.888185555828,31.7365416132748,-7.5));
#40745=CARTESIAN_POINT('Origin',(167.888185555828,31.7365416132748,-7.5));
#40746=CARTESIAN_POINT('Origin',(-42.86,-7.88821621745207,-7.5));
#40747=CARTESIAN_POINT('Origin',(-42.86,-7.88821621745207,-7.5));
#40748=CARTESIAN_POINT('Origin',(169.138185555828,29.5714781038137,-7.5));
#40749=CARTESIAN_POINT('Origin',(166.815861570388,28.6458370790927,-7.5));
#40750=CARTESIAN_POINT('Origin',(-42.86,-0.448216217452066,-7.5));
#40751=CARTESIAN_POINT('Origin',(-42.86,6.99178378254793,-7.5));
#40752=CARTESIAN_POINT('Origin',(168.742410169938,23.8123542251956,-7.5));
#40753=CARTESIAN_POINT('Origin',(152.4,6.99178378254796,-7.5));
#40754=CARTESIAN_POINT('Origin',(178.67101532033,35.0752599344873,7.5));
#40755=CARTESIAN_POINT('Origin',(177.42101532033,37.2403234439484,7.5));
#40756=CARTESIAN_POINT('Origin',(-4.10936255907258,-67.5662890908191,7.5));
#40757=CARTESIAN_POINT('Origin',(167.888185555828,31.7365416132748,7.5));
#40758=CARTESIAN_POINT('Origin',(-42.86,-7.88821621745207,7.5));
#40759=CARTESIAN_POINT('Origin',(-42.86,-7.88821621745207,7.5));
#40760=CARTESIAN_POINT('Origin',(169.138185555828,29.5714781038137,7.5));
#40761=CARTESIAN_POINT('Origin',(166.815861570388,28.6458370790927,7.5));
#40762=CARTESIAN_POINT('Origin',(-42.86,-0.448216217452066,7.5));
#40763=CARTESIAN_POINT('Origin',(-42.86,6.99178378254793,7.5));
#40764=CARTESIAN_POINT('Origin',(148.078108595041,75.6566458113737,7.5));
#40765=CARTESIAN_POINT('Origin',(-42.86,6.99178378254793,7.5));
#40798=UNCERTAINTY_MEASURE_WITH_UNIT(LENGTH_MEASURE(0.01),#40810,
'DISTANCE_ACCURACY_VALUE',
'Maximum model space distance between geometric entities at asserted c
onnectivities');
#40799=UNCERTAINTY_MEASURE_WITH_UNIT(LENGTH_MEASURE(0.01),#40810,
'DISTANCE_ACCURACY_VALUE',
'Maximum model space distance between geometric entities at asserted c
onnectivities');
#40808=(
GEOMETRIC_REPRESENTATION_CONTEXT(3)
GLOBAL_UNCERTAINTY_ASSIGNED_CONTEXT((#40798))
GLOBAL_UNIT_ASSIGNED_CONTEXT((#40810,#40812,#40813))
REPRESENTATION_CONTEXT('','3D')
);
#40809=(
GEOMETRIC_REPRESENTATION_CONTEXT(3)
GLOBAL_UNCERTAINTY_ASSIGNED_CONTEXT((#40799))
GLOBAL_UNIT_ASSIGNED_CONTEXT((#40810,#40812,#40813))
REPRESENTATION_CONTEXT('','3D')
);
#40810=(
LENGTH_UNIT()
NAMED_UNIT(*)
SI_UNIT(.MILLI.,.METRE.)
);
#40812=(
NAMED_UNIT(*)
PLANE_ANGLE_UNIT()
SI_UNIT($,.RADIAN.)
);
#40813=(
NAMED_UNIT(*)
SI_UNIT($,.STERADIAN.)
SOLID_ANGLE_UNIT()
);
#40822=SHAPE_DEFINITION_REPRESENTATION(#40831,#40864);
#40831=PRODUCT_DEFINITION_SHAPE('',$,#40874);
#40864=SHAPE_REPRESENTATION('',(#7055),#40808);
#40865=PRODUCT_DEFINITION_CONTEXT('part definition',#40894,'design');
#40874=PRODUCT_DEFINITION('Puller Link','Puller Link',#40883,#40865);
#40883=PRODUCT_DEFINITION_FORMATION('',$,#40904);
#40894=APPLICATION_CONTEXT(
'Core Data for Automotive Mechanical Design Process');
#40895=PRODUCT_CONTEXT('part definition',#40894,'mechanical');
#40904=PRODUCT('Puller Link','Puller Link',$,(#40895));
#40906=PRESENTATION_STYLE_ASSIGNMENT((#40911));
#40911=SURFACE_STYLE_USAGE(.BOTH.,#40916);
#40916=SURFACE_SIDE_STYLE('',(#40921));
#40921=SURFACE_STYLE_FILL_AREA(#40926);
#40926=FILL_AREA_STYLE('Opaque(227,224,212)',(#40931));
#40931=FILL_AREA_STYLE_COLOUR('Opaque(227,224,212)',#40936);
#40936=COLOUR_RGB('Opaque(227,224,212)',0.890196078431372,0.87843137254902,
0.831372549019608);
ENDSEC;
END-ISO-10303-21;
